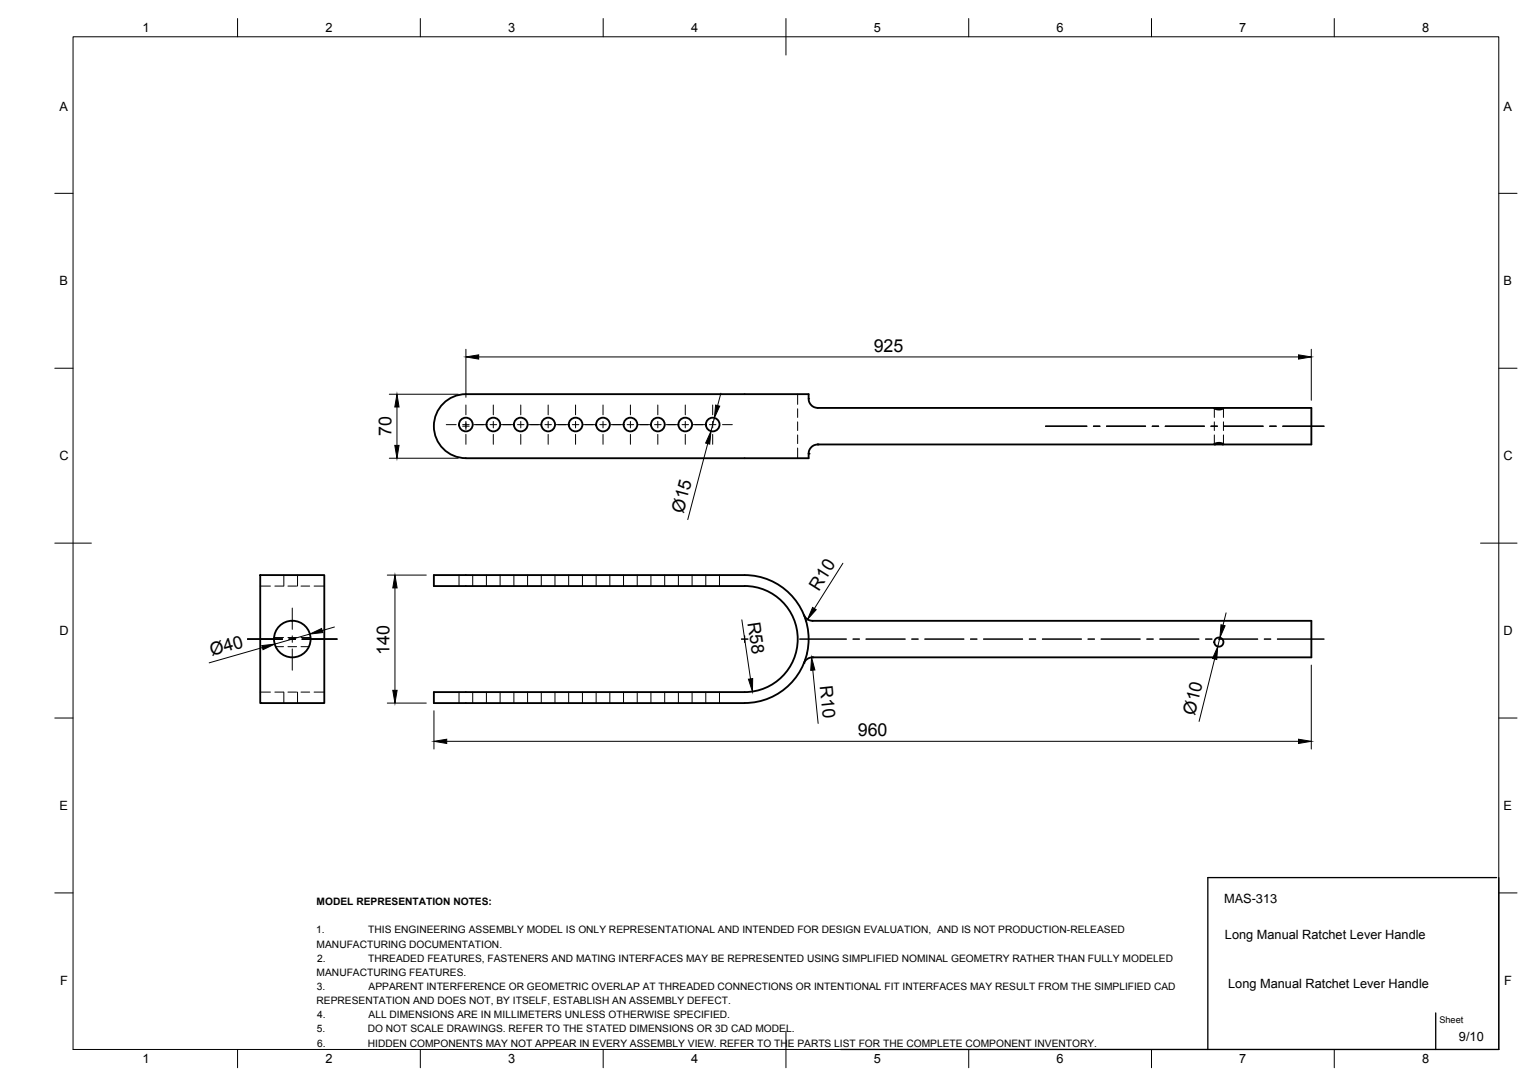
ISO-10303-21;
HEADER;
FILE_DESCRIPTION (('STEP AP214'),
    '1' );
FILE_NAME ('Long Manual Ratchet Lever Handle.step',
    '2026-10-06T09:36:00',
    ( '' ),
    ( '' ),
    'SwSTEP 2.0',
    'SolidWorks 2025',
    '' );
FILE_SCHEMA (( 'AUTOMOTIVE_DESIGN' ));
ENDSEC;

DATA;
#3=LINE ( 'NONE', #10333, #7200 ) ;
#5=EDGE_LOOP ( 'NONE', ( #11080, #1788 ) ) ;
#6=CARTESIAN_POINT ( 'NONE',  ( -384.9774416452893888, 80.69083648313058177, -144.6406486762352870 ) ) ;
#8=CARTESIAN_POINT ( 'NONE',  ( -374.9348459032029837, 78.20628728207141478, -105.0188168623670322 ) ) ;
#9=CARTESIAN_POINT ( 'NONE',  ( -305.0000000000000568, 81.99999999999995737, -89.68077099980384048 ) ) ;
#12=DIRECTION ( 'NONE',  ( -8.163404592832030268E-17, 1.000000000000000000, -0.000000000000000000 ) ) ;
#21=CARTESIAN_POINT ( 'NONE',  ( -824.1603064692799308, 83.67418067986842800, -144.6105757924095485 ) ) ;
#22=ADVANCED_FACE ( 'NONE', ( #9876 ), #2276, .F. ) ;
#24=CARTESIAN_POINT ( 'NONE',  ( -374.1619648394964770, 92.84764663444484256, -97.33358173750130504 ) ) ;
#35=CARTESIAN_POINT ( 'NONE',  ( -374.8624431792070482, 77.47276654782569949, -154.2594059479313842 ) ) ;
#36=CARTESIAN_POINT ( 'NONE',  ( -372.1683858186218004, 101.7385701426550071, -104.8071179324957569 ) ) ;
#42=LINE ( 'NONE', #11363, #8844 ) ;
#43=AXIS2_PLACEMENT_3D ( 'NONE', #1624, #5382, #1881 ) ;
#51=CARTESIAN_POINT ( 'NONE',  ( -379.1625717519825685, 101.9990905548760622, -123.9924296326342414 ) ) ;
#53=DIRECTION ( 'NONE',  ( -8.163404592832030268E-17, 1.000000000000000000, -0.000000000000000000 ) ) ;
#57=CARTESIAN_POINT ( 'NONE',  ( -370.6528479074003144, 106.2912024161782654, -136.2244394883228154 ) ) ;
#65=CARTESIAN_POINT ( 'NONE',  ( -365.0000000000000568, 81.99999999999997158, -124.6807709998038405 ) ) ;
#66=CARTESIAN_POINT ( 'NONE',  ( -119.9999999999999858, 12.00000000000001421, -126.4213562373086575 ) ) ;
#70=CARTESIAN_POINT ( 'NONE',  ( -384.9468357058332799, 80.02786880483864707, -144.5860799529720566 ) ) ;
#72=CARTESIAN_POINT ( 'NONE',  ( -374.8121035591796044, 76.80383275076532357, -95.25780428797004618 ) ) ;
#80=CARTESIAN_POINT ( 'NONE',  ( -97.49999999999998579, 24.00000000000001421, -126.4213562373088564 ) ) ;
#84=CARTESIAN_POINT ( 'NONE',  ( -384.0214413967224800, 73.66668219692796526, -106.4901515991773522 ) ) ;
#86=EDGE_CURVE ( 'NONE', #586, #9244, #5121, .T. ) ;
#90=VERTEX_POINT ( 'NONE', #4259 ) ;
#92=LINE ( 'NONE', #10358, #965 ) ;
#102=CARTESIAN_POINT ( 'NONE',  ( -383.2436296729866285, 93.11778785828077787, -108.0524282450768681 ) ) ;
#105=EDGE_CURVE ( 'NONE', #546, #9394, #11040, .T. ) ;
#111=DIRECTION ( 'NONE',  ( -8.163404592832030268E-17, 1.000000000000000000, -0.000000000000000000 ) ) ;
#120=EDGE_CURVE ( 'NONE', #2594, #3971, #5709, .T. ) ;
#121=EDGE_CURVE ( 'NONE', #609, #1988, #8932, .T. ) ;
#124=ORIENTED_EDGE ( 'NONE', *, *, #7991, .T. ) ;
#128=FACE_BOUND ( 'NONE', #2869, .T. ) ;
#130=CARTESIAN_POINT ( 'NONE',  ( -383.8870708247850985, 73.11411249519194655, -142.6104777306848916 ) ) ;
#132=CARTESIAN_POINT ( 'NONE',  ( -384.9021618238296583, 79.34260306531722051, -104.8553288783483453 ) ) ;
#141=CARTESIAN_POINT ( 'NONE',  ( -385.0078061158059768, 82.93686821115872476, -104.6668923901645769 ) ) ;
#143=EDGE_LOOP ( 'NONE', ( #3113, #5997, #4149, #12106, #10278, #5170, #6052 ) ) ;
#145=ORIENTED_EDGE ( 'NONE', *, *, #5842, .F. ) ;
#149=FACE_OUTER_BOUND ( 'NONE', #6887, .T. ) ;
#150=CIRCLE ( 'NONE', #8476, 7.500000000000007105 ) ;
#152=ORIENTED_EDGE ( 'NONE', *, *, #2859, .F. ) ;
#153=CARTESIAN_POINT ( 'NONE',  ( -374.9443013845391874, 79.15238586648754904, -154.5107090977903113 ) ) ;
#161=EDGE_CURVE ( 'NONE', #6627, #7697, #6700, .T. ) ;
#164=CARTESIAN_POINT ( 'NONE',  ( -150.0000000000000000, -9.213203435596451385, -126.4213562373084301 ) ) ;
#165=EDGE_CURVE ( 'NONE', #7498, #4712, #7501, .T. ) ;
#170=CARTESIAN_POINT ( 'NONE',  ( -371.2169330467067994, 104.7056300760318379, -109.5948443055706036 ) ) ;
#172=CARTESIAN_POINT ( 'NONE',  ( 1.414009460465297036E-14, -9.213203435596451385, -126.4213562373094959 ) ) ;
#174=CARTESIAN_POINT ( 'NONE',  ( -240.0000000000000000, 151.9999999999999716, -126.4213562373078190 ) ) ;
#179=ORIENTED_EDGE ( 'NONE', *, *, #161, .T. ) ;
#180=CYLINDRICAL_SURFACE ( 'NONE', #1475, 20.00000000000004619 ) ;
#181=CARTESIAN_POINT ( 'NONE',  ( -380.7070114274824846, 99.23877955377430737, -134.8374997946181111 ) ) ;
#183=EDGE_LOOP ( 'NONE', ( #1625, #2228, #7810, #4343, #5772, #11900, #7059 ) ) ;
#185=CARTESIAN_POINT ( 'NONE',  ( -384.7087986609971608, 86.59177257609081835, -144.1578396759514646 ) ) ;
#187=CARTESIAN_POINT ( 'NONE',  ( -382.1259332444888628, 67.82440028630135487, -110.5571689112878033 ) ) ;
#192=VERTEX_POINT ( 'NONE', #5981 ) ;
#200=CARTESIAN_POINT ( 'NONE',  ( -384.9575332945760806, 80.23676698716798228, -104.7563694268733059 ) ) ;
#204=CARTESIAN_POINT ( 'NONE',  ( -305.0000000000000568, 11.99999999999998224, -89.68077099980384048 ) ) ;
#210=DIRECTION ( 'NONE',  ( 3.061276722312011504E-17, -1.000000000000000000, 0.000000000000000000 ) ) ;
#211=CARTESIAN_POINT ( 'NONE',  ( -240.0000000000000000, 24.00000000000000711, -126.4213562373078190 ) ) ;
#218=EDGE_LOOP ( 'NONE', ( #11467, #11457 ) ) ;
#223=CIRCLE ( 'NONE', #7140, 7.500000000000007105 ) ;
#227=CARTESIAN_POINT ( 'NONE',  ( -820.5194676126008062, 82.43685310047841597, -104.6842045117117266 ) ) ;
#232=FACE_BOUND ( 'NONE', #2861, .T. ) ;
#233=VERTEX_POINT ( 'NONE', #6533 ) ;
#243=CARTESIAN_POINT ( 'NONE',  ( -383.7609474437092558, 91.40550212013970111, -142.3698073093449636 ) ) ;
#247=CARTESIAN_POINT ( 'NONE',  ( -384.0991065115986771, 74.01283611578425337, -143.0196247845297819 ) ) ;
#250=EDGE_LOOP ( 'NONE', ( #6658, #11800 ) ) ;
#263=ORIENTED_EDGE ( 'NONE', *, *, #5400, .T. ) ;
#270=ADVANCED_FACE ( 'NONE', ( #2701 ), #10246, .F. ) ;
#273=DIRECTION ( 'NONE',  ( -0.000000000000000000, -0.000000000000000000, -1.000000000000000000 ) ) ;
#283=EDGE_LOOP ( 'NONE', ( #6385, #2027 ) ) ;
#286=( BOUNDED_SURFACE ( )  B_SPLINE_SURFACE ( 3, 2, ( 
 ( #5085, #8801, #7187 ),
 ( #2485, #10957, #1263 ),
 ( #8857, #5024, #11650 ),
 ( #3170, #3727, #4408 ),
 ( #11016, #2547, #5517 ),
 ( #8178, #6322, #5324 ),
 ( #7317, #11945, #8318 ),
 ( #10089, #8249, #6509 ),
 ( #10030, #9093, #12007 ),
 ( #1688, #3526, #11218 ),
 ( #7251, #4472, #11082 ),
 ( #5581, #9355, #1623 ),
 ( #9160, #4606, #10151 ),
 ( #5381, #7377, #6262 ),
 ( #2741, #696, #632 ),
 ( #2607, #12145, #10219 ),
 ( #3462, #6382, #1561 ),
 ( #4667, #11150, #5445 ),
 ( #8445, #833, #9293 ),
 ( #9226, #767, #1818 ),
 ( #10279, #4542, #12077 ),
 ( #3587, #2673, #8382 ),
 ( #6448, #1756, #3659 ),
 ( #12203, #7433, #7499 ),
 ( #11272, #899, #10395 ),
 ( #1013, #1880, #10338 ),
 ( #9532, #6744, #8677 ),
 ( #2057, #5700, #5878 ),
 ( #7805, #8611, #130 ),
 ( #6810, #3848, #247 ),
 ( #5644, #3967, #9417 ),
 ( #1077, #4724, #2801 ),
 ( #8500, #5755, #10464 ),
 ( #4780, #6573, #7557 ),
 ( #9594, #5816, #8551 ),
 ( #2982, #6688, #4890 ),
 ( #953, #2119, #70 ),
 ( #1999, #7621, #6 ),
 ( #8730, #4035, #11511 ),
 ( #3782, #3908, #1938 ),
 ( #4834, #1139, #9657 ),
 ( #11329, #7682, #11389 ),
 ( #2928, #10521, #2870 ),
 ( #6630, #11451, #1198 ),
 ( #7737, #9474, #185 ),
 ( #10581, #3039, #4953 ),
 ( #11376, #2915, #12133 ),
 ( #2729, #1924, #3713 ),
 ( #5746, #7490, #5685 ),
 ( #6437, #6677, #10272 ),
 ( #11264, #5568, #10208 ),
 ( #9521, #1746, #2791 ),
 ( #8368, #11315, #11205 ),
 ( #3646, #5508, #1066 ),
 ( #9283, #5631, #1805 ),
 ( #6561, #1501, #821 ),
 ( #6498, #10325, #12064 ),
 ( #4766, #9405, #2854 ),
 ( #7611, #4713, #3773 ),
 ( #6620, #999, #8541 ),
 ( #57, #3836, #398 ),
 ( #9872, #8599, #11437 ) ),
 .UNSPECIFIED., .F., .F., .F. ) 
 B_SPLINE_SURFACE_WITH_KNOTS ( ( 4, 2, 2, 2, 2, 2, 2, 2, 2, 2, 2, 2, 2, 2, 2, 2, 2, 2, 2, 2, 2, 2, 2, 2, 2, 2, 2, 2, 2, 2, 4 ),
 ( 3, 3 ),
 ( 0.09449389133479987879, 0.1003997595432298551, 0.1063056277516598314, 0.1092585618558748195, 0.1107350289079823136, 0.1122114959600898076, 0.1181173641685197701, 0.1195938312206272502, 0.1210702982727347443, 0.1240232323769497325, 0.1269761664811647206, 0.1284526335332722147, 0.1299291005853797087, 0.1358349687938096850, 0.1387879028980246732, 0.1402643699501321672, 0.1417408370022396613, 0.1476467052106696376, 0.1491231722627771317, 0.1505996393148846257, 0.1535525734190996139, 0.1565055075233146020, 0.1594584416275295902, 0.1653643098359595387, 0.1683172439401744991, 0.1697937109922819932, 0.1712701780443894872, 0.1771760462528194635, 0.1801289803570344517, 0.1830819144612494398, 0.1889877826696794161 ),
 ( 0.000000000000000000, 1.000000000000000000 ),
 .UNSPECIFIED. ) 
 GEOMETRIC_REPRESENTATION_ITEM ( )  RATIONAL_B_SPLINE_SURFACE ( (
 ( 1.000000000000000000, 0.8172789612915526414, 1.000000000000000000),
 ( 1.000000000000000000, 0.8218272198189814359, 1.000000000000000000),
 ( 1.000000000000000000, 0.8252177520338900285, 1.000000000000000000),
 ( 1.000000000000000000, 0.8291640623197805704, 1.000000000000000000),
 ( 1.000000000000000000, 0.8296443862460527452, 1.000000000000000000),
 ( 1.000000000000000000, 0.8281763619574273871, 1.000000000000000000),
 ( 1.000000000000000000, 0.8273214979613470188, 1.000000000000000000),
 ( 1.000000000000000000, 0.8254906886306150327, 1.000000000000000000),
 ( 1.000000000000000000, 0.8247876722294519292, 1.000000000000000000),
 ( 1.000000000000000000, 0.8232192861295574149, 1.000000000000000000),
 ( 1.000000000000000000, 0.8223523569020266821, 1.000000000000000000),
 ( 1.000000000000000000, 0.8176244427683647675, 1.000000000000000000),
 ( 1.000000000000000000, 0.8125861978211987857, 1.000000000000000000),
 ( 1.000000000000000000, 0.8050068216217169947, 1.000000000000000000),
 ( 1.000000000000000000, 0.8034229420457332793, 1.000000000000000000),
 ( 1.000000000000000000, 0.8001526181735703069, 1.000000000000000000),
 ( 1.000000000000000000, 0.7984703186739749992, 1.000000000000000000),
 ( 1.000000000000000000, 0.7932997541396797914, 1.000000000000000000),
 ( 1.000000000000000000, 0.7896878191176920359, 1.000000000000000000),
 ( 1.000000000000000000, 0.7822263873999749650, 1.000000000000000000),
 ( 1.000000000000000000, 0.7783766572002538409, 1.000000000000000000),
 ( 1.000000000000000000, 0.7724948447777896243, 1.000000000000000000),
 ( 1.000000000000000000, 0.7705164146871855690, 1.000000000000000000),
 ( 1.000000000000000000, 0.7665366243600161278, 1.000000000000000000),
 ( 1.000000000000000000, 0.7645334732995007210, 1.000000000000000000),
 ( 1.000000000000000000, 0.7545994289160806723, 1.000000000000000000),
 ( 1.000000000000000000, 0.7468282588146691880, 1.000000000000000000),
 ( 1.000000000000000000, 0.7361158826353683127, 1.000000000000000000),
 ( 1.000000000000000000, 0.7327031703348744207, 1.000000000000000000),
 ( 1.000000000000000000, 0.7279177720675241714, 1.000000000000000000),
 ( 1.000000000000000000, 0.7263769756471946115, 1.000000000000000000),
 ( 1.000000000000000000, 0.7234575735669767083, 1.000000000000000000),
 ( 1.000000000000000000, 0.7220742453523991689, 1.000000000000000000),
 ( 1.000000000000000000, 0.7155655556167423992, 1.000000000000000000),
 ( 1.000000000000000000, 0.7116656400988581321, 1.000000000000000000),
 ( 1.000000000000000000, 0.7088249914908492100, 1.000000000000000000),
 ( 1.000000000000000000, 0.7083584775623817942, 1.000000000000000000),
 ( 1.000000000000000000, 0.7076383381209198076, 1.000000000000000000),
 ( 1.000000000000000000, 0.7073855737940044630, 1.000000000000000000),
 ( 1.000000000000000000, 0.7069609716970313151, 1.000000000000000000),
 ( 1.000000000000000000, 0.7071175024107954066, 1.000000000000000000),
 ( 1.000000000000000000, 0.7082797836801750790, 1.000000000000000000),
 ( 1.000000000000000000, 0.7092855318707916856, 1.000000000000000000),
 ( 1.000000000000000000, 0.7121081611133525113, 1.000000000000000000),
 ( 1.000000000000000000, 0.7139297788701386427, 1.000000000000000000),
 ( 1.000000000000000000, 0.7205123102341589592, 1.000000000000000000),
 ( 1.000000000000000000, 0.7262634879477153360, 1.000000000000000000),
 ( 1.000000000000000000, 0.7362377633225355433, 1.000000000000000000),
 ( 1.000000000000000000, 0.7397880641819555292, 1.000000000000000000),
 ( 1.000000000000000000, 0.7453704836958430224, 1.000000000000000000),
 ( 1.000000000000000000, 0.7472719429557758142, 1.000000000000000000),
 ( 1.000000000000000000, 0.7511059034608574825, 1.000000000000000000),
 ( 1.000000000000000000, 0.7530430930858292848, 1.000000000000000000),
 ( 1.000000000000000000, 0.7627925276597339321, 1.000000000000000000),
 ( 1.000000000000000000, 0.7707906794718482058, 1.000000000000000000),
 ( 1.000000000000000000, 0.7824407450661361452, 1.000000000000000000),
 ( 1.000000000000000000, 0.7862798113962640167, 1.000000000000000000),
 ( 1.000000000000000000, 0.7935920352645898790, 1.000000000000000000),
 ( 1.000000000000000000, 0.7970830763616314485, 1.000000000000000000),
 ( 1.000000000000000000, 0.8069453338637414541, 1.000000000000000000),
 ( 1.000000000000000000, 0.8127078027066928501, 1.000000000000000000),
 ( 1.000000000000000000, 0.8173438319342977154, 1.000000000000000000) ) ) 
 REPRESENTATION_ITEM ( '' )  SURFACE ( )  );
#288=AXIS2_PLACEMENT_3D ( 'NONE', #7289, #5491, #4381 ) ;
#290=CARTESIAN_POINT ( 'NONE',  ( -821.1548363108382773, 74.44610204637874062, -143.1996371447159788 ) ) ;
#294=CARTESIAN_POINT ( 'NONE',  ( -372.7969387542311210, 100.6399613739977497, -117.3710749709770198 ) ) ;
#297=FACE_BOUND ( 'NONE', #8922, .T. ) ;
#301=CARTESIAN_POINT ( 'NONE',  ( 7.500000000000022204, -9.213203435596451385, -126.4213562373094959 ) ) ;
#304=ORIENTED_EDGE ( 'NONE', *, *, #9166, .F. ) ;
#308=FACE_BOUND ( 'NONE', #6793, .T. ) ;
#311=DIRECTION ( 'NONE',  ( -1.000000000000000000, 0.000000000000000000, 0.000000000000000000 ) ) ;
#314=AXIS2_PLACEMENT_3D ( 'NONE', #7746, #6638, #6880 ) ;
#316=EDGE_LOOP ( 'NONE', ( #9146, #634 ) ) ;
#322=ORIENTED_EDGE ( 'NONE', *, *, #4849, .T. ) ;
#323=CYLINDRICAL_SURFACE ( 'NONE', #3336, 7.500000000000007105 ) ;
#324=CARTESIAN_POINT ( 'NONE',  ( -380.4203626278499542, 64.21146706504150359, -115.5204214313296376 ) ) ;
#330=DIRECTION ( 'NONE',  ( -1.000000000000000000, 0.000000000000000000, 0.000000000000000000 ) ) ;
#334=CIRCLE ( 'NONE', #5074, 57.99999999999999289 ) ;
#339=LINE ( 'NONE', #9047, #1075 ) ;
#342=EDGE_CURVE ( 'NONE', #12110, #8166, #11773, .T. ) ;
#351=AXIS2_PLACEMENT_3D ( 'NONE', #10311, #1910, #9449 ) ;
#352=DIRECTION ( 'NONE',  ( 0.000000000000000000, 0.000000000000000000, 1.000000000000000000 ) ) ;
#357=CIRCLE ( 'NONE', #7273, 7.499999999999992895 ) ;
#359=FACE_OUTER_BOUND ( 'NONE', #1203, .T. ) ;
#363=CARTESIAN_POINT ( 'NONE',  ( -375.0000000000000000, 81.99999999999995737, -89.68077099980384048 ) ) ;
#364=CARTESIAN_POINT ( 'NONE',  ( -374.9435208796285224, 79.09557628031252818, -94.85325544560421918 ) ) ;
#369=CARTESIAN_POINT ( 'NONE',  ( -90.00000000000000000, 152.0000000000000000, -126.4213562373088564 ) ) ;
#370=FACE_BOUND ( 'NONE', #3925, .T. ) ;
#373=CARTESIAN_POINT ( 'NONE',  ( -22.49999999999997868, -9.213203435596451385, -126.4213562373092685 ) ) ;
#379=ORIENTED_EDGE ( 'NONE', *, *, #11461, .F. ) ;
#380=ORIENTED_EDGE ( 'NONE', *, *, #161, .F. ) ;
#391=EDGE_CURVE ( 'NONE', #7319, #11283, #7095, .T. ) ;
#396=ORIENTED_EDGE ( 'NONE', *, *, #11359, .T. ) ;
#398=CARTESIAN_POINT ( 'NONE',  ( -380.0318359341034693, 100.5075656702939142, -132.3766003259852084 ) ) ;
#400=CYLINDRICAL_SURFACE ( 'NONE', #7484, 7.500000000000007105 ) ;
#401=EDGE_CURVE ( 'NONE', #10520, #8134, #578, .T. ) ;
#402=CARTESIAN_POINT ( 'NONE',  ( -180.0000000000000000, 12.00000000000001421, -126.4213562373082453 ) ) ;
#414=EDGE_CURVE ( 'NONE', #957, #11231, #4747, .T. ) ;
#419=CARTESIAN_POINT ( 'NONE',  ( -373.3204616456844747, 97.25197993938448349, -149.1095482086399784 ) ) ;
#442=CARTESIAN_POINT ( 'NONE',  ( -90.00000000000000000, 139.9999999999999716, -126.4213562373088564 ) ) ;
#448=DIRECTION ( 'NONE',  ( -1.000000000000000000, 0.000000000000000000, 0.000000000000000000 ) ) ;
#449=AXIS2_PLACEMENT_3D ( 'NONE', #6036, #2435, #448 ) ;
#451=CIRCLE ( 'NONE', #3416, 7.500000000000007105 ) ;
#466=CARTESIAN_POINT ( 'NONE',  ( -824.1545993022709808, 83.67440335600066703, -104.7509849144497736 ) ) ;
#469=LINE ( 'NONE', #4263, #6510 ) ;
#475=VECTOR ( 'NONE', #10063, 1000.000000000000000 ) ;
#478=ADVANCED_FACE ( 'NONE', ( #7705, #4803, #8575, #5910, #10363, #9558, #10543, #5725, #8699, #6657, #2827 ), #11414, .F. ) ;
#479=DIRECTION ( 'NONE',  ( 1.000000000000000000, 1.486905836551548832E-16, -0.000000000000000000 ) ) ;
#483=CIRCLE ( 'NONE', #3067, 7.500000000000007105 ) ;
#488=CARTESIAN_POINT ( 'NONE',  ( -374.5655304648819879, 89.79463081985890938, -153.3305951811361751 ) ) ;
#495=VERTEX_POINT ( 'NONE', #7765 ) ;
#496=EDGE_CURVE ( 'NONE', #546, #9681, #11781, .T. ) ;
#501=CARTESIAN_POINT ( 'NONE',  ( -379.1619848709567577, 102.0000000000000284, -123.4679443962072725 ) ) ;
#503=AXIS2_PLACEMENT_3D ( 'NONE', #6514, #3590, #1821 ) ;
#514=CARTESIAN_POINT ( 'NONE',  ( -374.8923245633905026, 85.92087493068839876, -95.01038614168759011 ) ) ;
#516=DIRECTION ( 'NONE',  ( 1.000000000000000000, 0.000000000000000000, 0.000000000000000000 ) ) ;
#517=CARTESIAN_POINT ( 'NONE',  ( -374.9998907128388623, 83.71581840400844499, -94.68015511488202662 ) ) ;
#518=ORIENTED_EDGE ( 'NONE', *, *, #8104, .T. ) ;
#521=ORIENTED_EDGE ( 'NONE', *, *, #11514, .T. ) ;
#528=DIRECTION ( 'NONE',  ( -8.163404592832031500E-17, 1.000000000000000000, 0.000000000000000000 ) ) ;
#529=CARTESIAN_POINT ( 'NONE',  ( -119.9999999999999858, 24.00000000000001421, -126.4213562373086575 ) ) ;
#531=CARTESIAN_POINT ( 'NONE',  ( -819.1462522098552199, 76.91297450996658824, -144.0236343770278609 ) ) ;
#536=ORIENTED_EDGE ( 'NONE', *, *, #1166, .F. ) ;
#537=FACE_OUTER_BOUND ( 'NONE', #8170, .T. ) ;
#542=EDGE_CURVE ( 'NONE', #9452, #8983, #6330, .T. ) ;
#546=VERTEX_POINT ( 'NONE', #9798 ) ;
#551=CARTESIAN_POINT ( 'NONE',  ( -370.0721644750066730, 107.8006199747635492, -130.5475387910841221 ) ) ;
#553=ADVANCED_FACE ( 'NONE', ( #5206 ), #2432, .T. ) ;
#555=DIRECTION ( 'NONE',  ( -8.163404592832030268E-17, 1.000000000000000000, -0.000000000000000000 ) ) ;
#563=ORIENTED_EDGE ( 'NONE', *, *, #496, .T. ) ;
#568=AXIS2_PLACEMENT_3D ( 'NONE', #5738, #2909, #4137 ) ;
#578=CIRCLE ( 'NONE', #1190, 7.500000000000007105 ) ;
#582=DIRECTION ( 'NONE',  ( 1.776356839400250465E-15, 0.000000000000000000, 1.000000000000000000 ) ) ;
#586=VERTEX_POINT ( 'NONE', #7135 ) ;
#589=DIRECTION ( 'NONE',  ( 1.000000000000000000, 2.040851148208007875E-17, 0.000000000000000000 ) ) ;
#590=CARTESIAN_POINT ( 'NONE',  ( -89.99999999999998579, -9.213203435596451385, -126.4213562373088564 ) ) ;
#591=ORIENTED_EDGE ( 'NONE', *, *, #3649, .T. ) ;
#597=CARTESIAN_POINT ( 'NONE',  ( -828.7636281597782499, 77.85463023298294161, -144.2471423470011018 ) ) ;
#606=FACE_OUTER_BOUND ( 'NONE', #11571, .T. ) ;
#609=VERTEX_POINT ( 'NONE', #9044 ) ;
#619=ORIENTED_EDGE ( 'NONE', *, *, #2215, .T. ) ;
#620=DIRECTION ( 'NONE',  ( -8.163404592832030268E-17, 1.000000000000000000, -0.000000000000000000 ) ) ;
#629=AXIS2_PLACEMENT_3D ( 'NONE', #5807, #4770, #10387 ) ;
#632=CARTESIAN_POINT ( 'NONE',  ( -380.5094386830780877, 64.38196187857104746, -134.1524419411843212 ) ) ;
#633=CARTESIAN_POINT ( 'NONE',  ( -29.99999999999998579, -9.213203435596451385, -126.4213562373092685 ) ) ;
#634=ORIENTED_EDGE ( 'NONE', *, *, #105, .F. ) ;
#637=EDGE_LOOP ( 'NONE', ( #8862, #9287, #8745, #1050 ) ) ;
#642=DIRECTION ( 'NONE',  ( 1.000000000000000000, 0.000000000000000000, 0.000000000000000000 ) ) ;
#648=CARTESIAN_POINT ( 'NONE',  ( -379.7887390581964837, 110.4014878146373633, -134.3428354745942102 ) ) ;
#652=CARTESIAN_POINT ( 'NONE',  ( -59.99999999999998579, -9.213203435596451385, -126.4213562373090696 ) ) ;
#654=EDGE_CURVE ( 'NONE', #2078, #6153, #6149, .T. ) ;
#658=CARTESIAN_POINT ( 'NONE',  ( -828.3259789886573117, 76.46577308275197993, -105.4592182070448416 ) ) ;
#666=EDGE_LOOP ( 'NONE', ( #1393, #6344, #2255, #9869 ) ) ;
#696=CARTESIAN_POINT ( 'NONE',  ( -373.1983853544816725, 64.95592079649878769, -135.2209821354010728 ) ) ;
#697=CYLINDRICAL_SURFACE ( 'NONE', #6175, 7.499999999999992895 ) ;
#698=EDGE_LOOP ( 'NONE', ( #3165, #3081, #2133, #7527, #1551 ) ) ;
#700=AXIS2_PLACEMENT_3D ( 'NONE', #10293, #12095, #7515 ) ;
#708=EDGE_CURVE ( 'NONE', #4719, #2602, #5527, .T. ) ;
#719=CARTESIAN_POINT ( 'NONE',  ( -30.00000000000000000, 139.9999999999999716, -126.4213562373092685 ) ) ;
#726=CARTESIAN_POINT ( 'NONE',  ( -369.8747838094790268, 55.70677269066278825, -126.1647431307883522 ) ) ;
#728=DIRECTION ( 'NONE',  ( 1.000000000000000000, 0.000000000000000000, 0.000000000000000000 ) ) ;
#735=DIRECTION ( 'NONE',  ( 0.000000000000000000, 1.000000000000000000, -0.000000000000000000 ) ) ;
#741=DIRECTION ( 'NONE',  ( 1.000000000000000000, 1.486905836551548832E-16, -0.000000000000000000 ) ) ;
#758=ORIENTED_EDGE ( 'NONE', *, *, #1083, .F. ) ;
#767=CARTESIAN_POINT ( 'NONE',  ( -373.7506463163484796, 67.50546400631965582, -138.5607443211070802 ) ) ;
#774=DIRECTION ( 'NONE',  ( 3.061276722312011504E-17, -1.000000000000000000, 0.000000000000000000 ) ) ;
#784=CARTESIAN_POINT ( 'NONE',  ( -369.8980370199456047, 108.2344238686749520, -123.1401886717858787 ) ) ;
#785=ORIENTED_EDGE ( 'NONE', *, *, #9267, .F. ) ;
#787=VECTOR ( 'NONE', #1857, 1000.000000000000000 ) ;
#794=CARTESIAN_POINT ( 'NONE',  ( -820.7525053003647599, 74.71879621637245350, -106.0522004026985456 ) ) ;
#801=CARTESIAN_POINT ( 'NONE',  ( -374.4786324000669424, 91.82513850978268977, -107.1885437437087063 ) ) ;
#805=DIRECTION ( 'NONE',  ( -1.000000000000000000, 0.000000000000000000, 0.000000000000000000 ) ) ;
#817=CARTESIAN_POINT ( 'NONE',  ( -82.49999999999997158, -9.213203435596451385, -126.4213562373088564 ) ) ;
#818=VERTEX_POINT ( 'NONE', #8260 ) ;
#820=LINE ( 'NONE', #1865, #6878 ) ;
#821=CARTESIAN_POINT ( 'NONE',  ( -381.5603242327452449, 97.47709203580956228, -137.3647392459991750 ) ) ;
#824=EDGE_CURVE ( 'NONE', #11283, #7319, #1411, .T. ) ;
#828=AXIS2_PLACEMENT_3D ( 'NONE', #6958, #5155, #8814 ) ;
#833=CARTESIAN_POINT ( 'NONE',  ( -373.5661612086483387, 66.59315941246912018, -137.5313104353387530 ) ) ;
#836=DIRECTION ( 'NONE',  ( -1.000000000000000000, 0.000000000000000000, 0.000000000000000000 ) ) ;
#845=DIRECTION ( 'NONE',  ( 2.040851148208007875E-17, -1.000000000000000000, -0.000000000000000000 ) ) ;
#846=VECTOR ( 'NONE', #8160, 1000.000000000000000 ) ;
#847=CIRCLE ( 'NONE', #2211, 7.500000000000007105 ) ;
#849=ORIENTED_EDGE ( 'NONE', *, *, #4932, .F. ) ;
#851=CARTESIAN_POINT ( 'NONE',  ( -370.4631672708575252, 106.7912974028927806, -114.8027370444668662 ) ) ;
#855=CARTESIAN_POINT ( 'NONE',  ( -187.5000000000000000, 24.00000000000001421, -126.4213562373082453 ) ) ;
#859=AXIS2_PLACEMENT_3D ( 'NONE', #211, #8634, #7891 ) ;
#860=EDGE_CURVE ( 'NONE', #3022, #6536, #1699, .T. ) ;
#861=CARTESIAN_POINT ( 'NONE',  ( -823.4970567115291260, 73.67398878492905112, -106.4962298347509631 ) ) ;
#863=CARTESIAN_POINT ( 'NONE',  ( -826.3639150177590409, 74.35254223074673519, -143.1619793993633323 ) ) ;
#864=VERTEX_POINT ( 'NONE', #11160 ) ;
#865=CARTESIAN_POINT ( 'NONE',  ( -372.8682051073146226, 64.83784294256510350, -147.4127590854037635 ) ) ;
#866=CARTESIAN_POINT ( 'NONE',  ( -384.1845455826150442, 89.69765040021600555, -106.1749927342177102 ) ) ;
#876=LINE ( 'NONE', #8424, #1553 ) ;
#878=CARTESIAN_POINT ( 'NONE',  ( -369.9630775916107268, 108.0732521340322876, -120.6787736983387163 ) ) ;
#899=CARTESIAN_POINT ( 'NONE',  ( -374.1450238171013893, 69.75518729278782359, -140.5780087988560183 ) ) ;
#903=EDGE_CURVE ( 'NONE', #7035, #9732, #8909, .T. ) ;
#905=AXIS2_PLACEMENT_3D ( 'NONE', #9527, #2866, #1994 ) ;
#917=CARTESIAN_POINT ( 'NONE',  ( -373.0711960171485657, 98.34294693636040563, -101.1726803376526505 ) ) ;
#921=DIRECTION ( 'NONE',  ( 0.000000000000000000, -0.9464175275073136717, 0.3229456047493806103 ) ) ;
#922=CARTESIAN_POINT ( 'NONE',  ( -828.8285638327206470, 78.34605190446892209, -105.0145692953448133 ) ) ;
#925=EDGE_LOOP ( 'NONE', ( #10478, #7807, #5815, #9444 ) ) ;
#932=AXIS2_PLACEMENT_3D ( 'NONE', #9914, #5152, #9977 ) ;
#945=VECTOR ( 'NONE', #10974, 1000.000000000000000 ) ;
#946=ORIENTED_EDGE ( 'NONE', *, *, #12081, .T. ) ;
#952=MECHANICAL_DESIGN_GEOMETRIC_PRESENTATION_REPRESENTATION('',(#1937),#2926);
#953=CARTESIAN_POINT ( 'NONE',  ( -374.9534812425817449, 79.41157780634799224, -154.5387344296071319 ) ) ;
#957=VERTEX_POINT ( 'NONE', #3052 ) ;
#958=CIRCLE ( 'NONE', #351, 7.500000000000007105 ) ;
#960=CARTESIAN_POINT ( 'NONE',  ( -97.49999999999998579, -9.213203435596451385, -126.4213562373088564 ) ) ;
#965=VECTOR ( 'NONE', #2823, 1000.000000000000000 ) ;
#966=VERTEX_POINT ( 'NONE', #80 ) ;
#970=CARTESIAN_POINT ( 'NONE',  ( -369.9251870295186677, 108.1672116062914029, -127.1279719650820255 ) ) ;
#973=DIRECTION ( 'NONE',  ( -8.163404592832030268E-17, 1.000000000000000000, -0.000000000000000000 ) ) ;
#976=AXIS2_PLACEMENT_3D ( 'NONE', #9716, #10818, #2236 ) ;
#979=CARTESIAN_POINT ( 'NONE',  ( -150.0000000000000000, -9.213203435596451385, -126.4213562373084301 ) ) ;
#981=CARTESIAN_POINT ( 'NONE',  ( -210.0000000000000000, -9.213203435596478030, -126.4213562373080180 ) ) ;
#996=DIRECTION ( 'NONE',  ( -8.163404592832030268E-17, 1.000000000000000000, -0.000000000000000000 ) ) ;
#999=CARTESIAN_POINT ( 'NONE',  ( -373.1039460868908009, 99.45530451436835051, -134.6103044504524462 ) ) ;
#1011=FACE_BOUND ( 'NONE', #10350, .T. ) ;
#1013=CARTESIAN_POINT ( 'NONE',  ( -373.1558531919824873, 65.98301015230569533, -148.5292176372442725 ) ) ;
#1014=EDGE_CURVE ( 'NONE', #11690, #11084, #1599, .T. ) ;
#1017=CYLINDRICAL_SURFACE ( 'NONE', #5268, 7.499999999999992895 ) ;
#1018=AXIS2_PLACEMENT_3D ( 'NONE', #7016, #1338, #5969 ) ;
#1022=CYLINDRICAL_SURFACE ( 'NONE', #4880, 7.500000000000007994 ) ;
#1027=ORIENTED_EDGE ( 'NONE', *, *, #3586, .T. ) ;
#1029=CARTESIAN_POINT ( 'NONE',  ( -826.3405481598703091, 83.00984762678743323, -144.6560901833811670 ) ) ;
#1032=CARTESIAN_POINT ( 'NONE',  ( -370.7906933011090587, 105.9194442196002797, -112.1115210325544211 ) ) ;
#1044=AXIS2_PLACEMENT_3D ( 'NONE', #7346, #6420, #10190 ) ;
#1046=DIRECTION ( 'NONE',  ( 0.000000000000000000, 1.000000000000000000, -0.000000000000000000 ) ) ;
#1047=CARTESIAN_POINT ( 'NONE',  ( -373.3860983059685168, 96.94888192596226872, -100.0157719451421201 ) ) ;
#1050=ORIENTED_EDGE ( 'NONE', *, *, #6377, .F. ) ;
#1058=LINE ( 'NONE', #8589, #4412 ) ;
#1061=CARTESIAN_POINT ( 'NONE',  ( -379.2435172475073841, 101.8653349591487398, -122.0127727988336233 ) ) ;
#1062=DIRECTION ( 'NONE',  ( -8.163404592832031500E-17, 1.000000000000000000, 0.000000000000000000 ) ) ;
#1063=CARTESIAN_POINT ( 'NONE',  ( -187.5000000000000000, -9.213203435596478030, -126.4213562373082453 ) ) ;
#1064=ORIENTED_EDGE ( 'NONE', *, *, #2859, .T. ) ;
#1066=CARTESIAN_POINT ( 'NONE',  ( -382.5082707561835491, 95.24935193720608595, -139.7187524817161659 ) ) ;
#1073=DIRECTION ( 'NONE',  ( 1.000000000000000000, 8.163404592832031500E-17, 0.000000000000000000 ) ) ;
#1075=VECTOR ( 'NONE', #9864, 1000.000000000000000 ) ;
#1077=CARTESIAN_POINT ( 'NONE',  ( -374.3833522074543794, 72.72018747391939542, -152.7479631189390830 ) ) ;
#1078=DIRECTION ( 'NONE',  ( -1.000000000000000000, 0.000000000000000000, 0.000000000000000000 ) ) ;
#1079=CARTESIAN_POINT ( 'NONE',  ( -372.7333679680364753, 64.32814225526269070, -102.4919576850857936 ) ) ;
#1080=LINE ( 'NONE', #3911, #7467 ) ;
#1083=EDGE_CURVE ( 'NONE', #6536, #957, #334, .T. ) ;
#1084=VECTOR ( 'NONE', #3811, 1000.000000000000000 ) ;
#1090=ORIENTED_EDGE ( 'NONE', *, *, #6921, .F. ) ;
#1099=CARTESIAN_POINT ( 'NONE',  ( -119.9999999999999858, 12.00000000000001421, -126.4213562373086575 ) ) ;
#1107=ADVANCED_FACE ( 'NONE', ( #5426, #10197 ), #7355, .T. ) ;
#1108=ORIENTED_EDGE ( 'NONE', *, *, #8570, .F. ) ;
#1120=CARTESIAN_POINT ( 'NONE',  ( -379.3756478403909682, 101.6476682939905629, -120.7185890014945784 ) ) ;
#1121=EDGE_CURVE ( 'NONE', #818, #12110, #7480, .T. ) ;
#1123=CARTESIAN_POINT ( 'NONE',  ( -60.00000000000000000, 152.0000000000000000, -126.4213562373090696 ) ) ;
#1124=ORIENTED_EDGE ( 'NONE', *, *, #4496, .F. ) ;
#1128=DIRECTION ( 'NONE',  ( 0.000000000000000000, 0.000000000000000000, 1.000000000000000000 ) ) ;
#1132=DIRECTION ( 'NONE',  ( -8.163404592832030268E-17, 1.000000000000000000, -0.000000000000000000 ) ) ;
#1136=DIRECTION ( 'NONE',  ( -1.000000000000000000, -2.040851148208007875E-17, 0.000000000000000000 ) ) ;
#1138=ORIENTED_EDGE ( 'NONE', *, *, #11671, .T. ) ;
#1139=CARTESIAN_POINT ( 'NONE',  ( -374.9999469826531140, 82.55142442433661643, -144.6804108797159643 ) ) ;
#1151=ORIENTED_EDGE ( 'NONE', *, *, #496, .F. ) ;
#1152=FACE_OUTER_BOUND ( 'NONE', #3781, .T. ) ;
#1157=EDGE_LOOP ( 'NONE', ( #5522, #946 ) ) ;
#1166=EDGE_CURVE ( 'NONE', #7292, #12134, #2810, .T. ) ;
#1170=ORIENTED_EDGE ( 'NONE', *, *, #4570, .T. ) ;
#1190=AXIS2_PLACEMENT_3D ( 'NONE', #8519, #10425, #3809 ) ;
#1192=VERTEX_POINT ( 'NONE', #5559 ) ;
#1193=CARTESIAN_POINT ( 'NONE',  ( -142.5000000000000000, 24.00000000000001421, -126.4213562373084301 ) ) ;
#1195=CARTESIAN_POINT ( 'NONE',  ( -382.8391312933034669, 94.32133009973502169, -140.4452862510830755 ) ) ;
#1198=CARTESIAN_POINT ( 'NONE',  ( -384.7868575475719695, 85.94460086465754500, -144.2989652200420494 ) ) ;
#1200=CARTESIAN_POINT ( 'NONE',  ( -374.6039973053199788, 73.23368555401432900, -106.6028248502465061 ) ) ;
#1203=EDGE_LOOP ( 'NONE', ( #10575, #3913, #8610, #5820 ) ) ;
#1204=ORIENTED_EDGE ( 'NONE', *, *, #8707, .F. ) ;
#1208=EDGE_LOOP ( 'NONE', ( #11716, #6844, #396, #5185 ) ) ;
#1209=CARTESIAN_POINT ( 'NONE',  ( -384.5582068021247437, 87.62753060213235301, -105.4794641167554232 ) ) ;
#1212=EDGE_LOOP ( 'NONE', ( #8401, #12199, #1064, #4026 ) ) ;
#1222=VECTOR ( 'NONE', #11804, 1000.000000000000000 ) ;
#1229=EDGE_CURVE ( 'NONE', #6950, #4621, #9334, .T. ) ;
#1233=VERTEX_POINT ( 'NONE', #1916 ) ;
#1235=CARTESIAN_POINT ( 'NONE',  ( -819.4838385048373084, 81.17047855582150362, -104.6961160549175531 ) ) ;
#1250=FACE_BOUND ( 'NONE', #218, .T. ) ;
#1252=FACE_OUTER_BOUND ( 'NONE', #4826, .T. ) ;
#1260=DIRECTION ( 'NONE',  ( -8.163404592832030268E-17, 1.000000000000000000, -0.000000000000000000 ) ) ;
#1263=CARTESIAN_POINT ( 'NONE',  ( -379.5535208569121437, 62.65259614875188987, -119.4499276052048771 ) ) ;
#1275=DIRECTION ( 'NONE',  ( -1.000000000000000000, 0.000000000000000000, 0.000000000000000000 ) ) ;
#1276=UNCERTAINTY_MEASURE_WITH_UNIT (LENGTH_MEASURE( 1.000000000000000082E-05 ), #10584, 'distance_accuracy_value', 'NONE');
#1277=ADVANCED_FACE ( 'NONE', ( #8533 ), #3766, .F. ) ;
#1279=DIRECTION ( 'NONE',  ( -1.000000000000000000, 0.000000000000000000, 0.000000000000000000 ) ) ;
#1294=CARTESIAN_POINT ( 'NONE',  ( -305.0000000000000568, 81.99999999999995737, -89.68077099980384048 ) ) ;
#1295=CARTESIAN_POINT ( 'NONE',  ( -67.50000000000000000, 139.9999999999999716, -126.4213562373090696 ) ) ;
#1298=DIRECTION ( 'NONE',  ( 1.000000000000000000, 0.000000000000000000, 0.000000000000000000 ) ) ;
#1302=DIRECTION ( 'NONE',  ( 1.000000000000000000, 0.000000000000000000, -0.000000000000000000 ) ) ;
#1309=EDGE_LOOP ( 'NONE', ( #11192, #9487, #5444, #2692 ) ) ;
#1313=DIRECTION ( 'NONE',  ( 2.040851148208007875E-17, -1.000000000000000000, -0.000000000000000000 ) ) ;
#1316=EDGE_CURVE ( 'NONE', #9732, #7035, #847, .T. ) ;
#1318=ORIENTED_EDGE ( 'NONE', *, *, #10928, .F. ) ;
#1324=CIRCLE ( 'NONE', #7436, 7.500000000000007105 ) ;
#1325=FACE_OUTER_BOUND ( 'NONE', #1959, .T. ) ;
#1327=ORIENTED_EDGE ( 'NONE', *, *, #2177, .F. ) ;
#1338=DIRECTION ( 'NONE',  ( -1.000000000000000000, -1.486905836551548832E-16, 0.000000000000000000 ) ) ;
#1344=EDGE_CURVE ( 'NONE', #233, #4125, #7080, .T. ) ;
#1352=CARTESIAN_POINT ( 'NONE',  ( -826.0484035456422589, 83.16661265238070655, -104.7144245788473000 ) ) ;
#1354=CARTESIAN_POINT ( 'NONE',  ( -373.2899463707186669, 98.65819193945954169, -113.5174344538613411 ) ) ;
#1356=VECTOR ( 'NONE', #973, 1000.000000000000000 ) ;
#1358=DIRECTION ( 'NONE',  ( -8.163404592832030268E-17, 1.000000000000000000, -0.000000000000000000 ) ) ;
#1362=CARTESIAN_POINT ( 'NONE',  ( -374.6494996980943597, 74.87479940665586753, -95.76181135420617352 ) ) ;
#1364=CIRCLE ( 'NONE', #11242, 7.500000000000020428 ) ;
#1366=CARTESIAN_POINT ( 'NONE',  ( -383.3184125885782692, 71.07417258413192940, -141.4727867585951344 ) ) ;
#1368=CARTESIAN_POINT ( 'NONE',  ( -217.5000000000000000, 24.00000000000000711, -126.4213562373080180 ) ) ;
#1371=CARTESIAN_POINT ( 'NONE',  ( -210.0000000000000000, -9.213203435596478030, -126.4213562373080180 ) ) ;
#1373=AXIS2_PLACEMENT_3D ( 'NONE', #6165, #1466, #352 ) ;
#1380=DIRECTION ( 'NONE',  ( -1.000000000000000000, 0.000000000000000000, 0.000000000000000000 ) ) ;
#1385=ORIENTED_EDGE ( 'NONE', *, *, #6553, .F. ) ;
#1393=ORIENTED_EDGE ( 'NONE', *, *, #4461, .F. ) ;
#1395=CARTESIAN_POINT ( 'NONE',  ( -370.4431240880616656, 57.15653990293294839, -114.9924028573224035 ) ) ;
#1407=EDGE_CURVE ( 'NONE', #11206, #8134, #1058, .T. ) ;
#1408=ADVANCED_FACE ( 'NONE', ( #7660 ), #11430, .F. ) ;
#1411=CIRCLE ( 'NONE', #8337, 7.500000000000007105 ) ;
#1418=EDGE_CURVE ( 'NONE', #8166, #12110, #10504, .T. ) ;
#1420=CARTESIAN_POINT ( 'NONE',  ( -202.4999999999999716, 151.9999999999999716, -126.4213562373080180 ) ) ;
#1421=CARTESIAN_POINT ( 'NONE',  ( -374.0142209343122772, 70.27728921848439825, -97.82681790556920021 ) ) ;
#1427=CARTESIAN_POINT ( 'NONE',  ( -379.7840584701665421, 63.05619850801249981, -131.1209148564447275 ) ) ;
#1432=VECTOR ( 'NONE', #8423, 1000.000000000000000 ) ;
#1435=AXIS2_PLACEMENT_3D ( 'NONE', #5645, #4409, #4607 ) ;
#1439=DIRECTION ( 'NONE',  ( -1.000000000000000000, 0.000000000000000000, 0.000000000000000000 ) ) ;
#1441=CARTESIAN_POINT ( 'NONE',  ( -67.49999999999998579, 12.00000000000001421, -126.4213562373090696 ) ) ;
#1442=CIRCLE ( 'NONE', #9353, 7.500000000000007105 ) ;
#1447=ORIENTED_EDGE ( 'NONE', *, *, #5229, .T. ) ;
#1449=CARTESIAN_POINT ( 'NONE',  ( -372.7937968025706255, 63.34872752675727270, -117.4098597798456041 ) ) ;
#1451=CARTESIAN_POINT ( 'NONE',  ( -270.0000000000000000, 151.9999999999999716, -126.4213562373076059 ) ) ;
#1461=VECTOR ( 'NONE', #6301, 1000.000000000000000 ) ;
#1464=AXIS2_PLACEMENT_3D ( 'NONE', #6953, #10721, #7642 ) ;
#1466=DIRECTION ( 'NONE',  ( 0.000000000000000000, 1.000000000000000000, -0.000000000000000000 ) ) ;
#1467=CARTESIAN_POINT ( 'NONE',  ( -305.0000000000000568, 151.9999999999999716, -159.6807709998038547 ) ) ;
#1475=AXIS2_PLACEMENT_3D ( 'NONE', #65, #3902, #8672 ) ;
#1478=DIRECTION ( 'NONE',  ( -8.163404592832030268E-17, 1.000000000000000000, -0.000000000000000000 ) ) ;
#1479=CARTESIAN_POINT ( 'NONE',  ( -373.6864081855313202, 68.44581660449321703, -98.94085437915049397 ) ) ;
#1489=CYLINDRICAL_SURFACE ( 'NONE', #11185, 7.500000000000007105 ) ;
#1491=CARTESIAN_POINT ( 'NONE',  ( 0.000000000000000000, 152.0000000000000000, -89.68077099980384048 ) ) ;
#1492=CYLINDRICAL_SURFACE ( 'NONE', #11425, 35.00000000000000000 ) ;
#1497=EDGE_LOOP ( 'NONE', ( #11987, #7229, #521, #8305 ) ) ;
#1501=CARTESIAN_POINT ( 'NONE',  ( -373.7456202422138176, 96.52126932011218230, -138.5319469839025714 ) ) ;
#1502=FACE_OUTER_BOUND ( 'NONE', #6460, .T. ) ;
#1511=ORIENTED_EDGE ( 'NONE', *, *, #12140, .F. ) ;
#1512=CARTESIAN_POINT ( 'NONE',  ( -150.0000000000000000, 24.00000000000001421, -126.4213562373084301 ) ) ;
#1519=CIRCLE ( 'NONE', #9424, 35.00000000000000000 ) ;
#1524=DIRECTION ( 'NONE',  ( -8.163404592832030268E-17, 1.000000000000000000, -0.000000000000000000 ) ) ;
#1526=CARTESIAN_POINT ( 'NONE',  ( -820.7495229154725394, 74.72132575352334527, -143.3103177350645296 ) ) ;
#1530=LINE ( 'NONE', #11678, #9648 ) ;
#1531=DIRECTION ( 'NONE',  ( -3.061276722312011504E-17, 1.000000000000000000, -0.000000000000000000 ) ) ;
#1532=ORIENTED_EDGE ( 'NONE', *, *, #10312, .T. ) ;
#1535=DIRECTION ( 'NONE',  ( -1.000000000000000000, 0.000000000000000000, 0.000000000000000000 ) ) ;
#1537=CARTESIAN_POINT ( 'NONE',  ( -370.5981920676458685, 57.56502298018414621, -113.6242979122189922 ) ) ;
#1547=CARTESIAN_POINT ( 'NONE',  ( -363.0000000000000568, 81.99999999999995737, -89.68077099980384048 ) ) ;
#1550=DIRECTION ( 'NONE',  ( -1.000000000000000000, 0.000000000000000000, 0.000000000000000000 ) ) ;
#1551=ORIENTED_EDGE ( 'NONE', *, *, #2991, .T. ) ;
#1553=VECTOR ( 'NONE', #3704, 1000.000000000000000 ) ;
#1560=EDGE_CURVE ( 'NONE', #9452, #495, #3946, .T. ) ;
#1561=CARTESIAN_POINT ( 'NONE',  ( -380.7611941007019141, 64.86892148911482536, -135.0070643092065836 ) ) ;
#1562=CARTESIAN_POINT ( 'NONE',  ( -381.5042408296175722, 97.59833250969687413, -112.1498553144568717 ) ) ;
#1565=DIRECTION ( 'NONE',  ( 0.000000000000000000, 0.000000000000000000, 1.000000000000000000 ) ) ;
#1568=CARTESIAN_POINT ( 'NONE',  ( -180.0000000000000000, -9.213203435596478030, -126.4213562373082453 ) ) ;
#1569=AXIS2_PLACEMENT_3D ( 'NONE', #11542, #273, #10607 ) ;
#1573=CARTESIAN_POINT ( 'NONE',  ( 7.500000000000020428, 12.00000000000001776, -126.4213562373094959 ) ) ;
#1575=CARTESIAN_POINT ( 'NONE',  ( -385.0247828397638159, 81.99275599918267687, -104.6365852498861102 ) ) ;
#1584=DIRECTION ( 'NONE',  ( -0.000000000000000000, -0.000000000000000000, 1.000000000000000000 ) ) ;
#1597=ORIENTED_EDGE ( 'NONE', *, *, #6226, .T. ) ;
#1599=LINE ( 'NONE', #10711, #846 ) ;
#1607=ORIENTED_EDGE ( 'NONE', *, *, #8386, .T. ) ;
#1608=LINE ( 'NONE', #7425, #3319 ) ;
#1615=VERTEX_POINT ( 'NONE', #11629 ) ;
#1617=ORIENTED_EDGE ( 'NONE', *, *, #4280, .F. ) ;
#1623=CARTESIAN_POINT ( 'NONE',  ( -379.7747414317349808, 63.03754323421768646, -131.1733032197525119 ) ) ;
#1624=CARTESIAN_POINT ( 'NONE',  ( -59.99999999999998579, 24.00000000000001421, -126.4213562373090696 ) ) ;
#1625=ORIENTED_EDGE ( 'NONE', *, *, #7440, .F. ) ;
#1630=ADVANCED_FACE ( 'NONE', ( #6917 ), #5866, .T. ) ;
#1635=CARTESIAN_POINT ( 'NONE',  ( -384.9998751003590201, 83.30729021256857436, -104.6803604098840168 ) ) ;
#1637=DIRECTION ( 'NONE',  ( 0.000000000000000000, 0.9467162604879117982, -0.3220688158263456113 ) ) ;
#1647=DIRECTION ( 'NONE',  ( 1.000000000000000000, 0.000000000000000000, 0.000000000000000000 ) ) ;
#1649=CARTESIAN_POINT ( 'NONE',  ( -822.1849787629541879, 73.94083650471891644, -142.9856651621327046 ) ) ;
#1652=CARTESIAN_POINT ( 'NONE',  ( -370.0238914150202731, 56.07874637648789928, -129.5483826961032037 ) ) ;
#1660=AXIS2_PLACEMENT_3D ( 'NONE', #172, #6791, #5799 ) ;
#1677=ORIENTED_EDGE ( 'NONE', *, *, #12039, .T. ) ;
#1684=ORIENTED_EDGE ( 'NONE', *, *, #11803, .T. ) ;
#1686=EDGE_CURVE ( 'NONE', #192, #10150, #2698, .T. ) ;
#1688=CARTESIAN_POINT ( 'NONE',  ( -370.1689562966705580, 56.44580195161717029, -131.5601801359200920 ) ) ;
#1689=DIRECTION ( 'NONE',  ( -8.163404592832030268E-17, 1.000000000000000000, -0.000000000000000000 ) ) ;
#1699=LINE ( 'NONE', #7261, #4772 ) ;
#1704=EDGE_CURVE ( 'NONE', #6191, #9127, #4013, .T. ) ;
#1707=CARTESIAN_POINT ( 'NONE',  ( -82.49999999999998579, 152.0000000000000000, -126.4213562373088564 ) ) ;
#1708=VERTEX_POINT ( 'NONE', #11240 ) ;
#1712=ORIENTED_EDGE ( 'NONE', *, *, #6388, .F. ) ;
#1715=AXIS2_PLACEMENT_3D ( 'NONE', #7182, #3409, #3235 ) ;
#1717=CARTESIAN_POINT ( 'NONE',  ( -822.1919554870369211, 73.93830887977112809, -106.3769876045755467 ) ) ;
#1718=CARTESIAN_POINT ( 'NONE',  ( -826.9024563477383936, 74.71743289348825101, -143.3087845970614183 ) ) ;
#1719=ORIENTED_EDGE ( 'NONE', *, *, #8523, .F. ) ;
#1723=CARTESIAN_POINT ( 'NONE',  ( -374.0275851353517851, 95.01260271039970462, -109.3552309949570400 ) ) ;
#1726=EDGE_CURVE ( 'NONE', #5232, #609, #4808, .T. ) ;
#1730=CARTESIAN_POINT ( 'NONE',  ( -22.49999999999999289, 139.9999999999999716, -126.4213562373092685 ) ) ;
#1736=CIRCLE ( 'NONE', #11795, 7.500000000000007994 ) ;
#1744=ORIENTED_EDGE ( 'NONE', *, *, #860, .F. ) ;
#1746=CARTESIAN_POINT ( 'NONE',  ( -374.4050532074698481, 92.42149850801368416, -141.8266576912406833 ) ) ;
#1755=ORIENTED_EDGE ( 'NONE', *, *, #4932, .T. ) ;
#1756=CARTESIAN_POINT ( 'NONE',  ( -374.0178982243409109, 68.97857190266184091, -139.9467288357900827 ) ) ;
#1760=VECTOR ( 'NONE', #8649, 1000.000000000000000 ) ;
#1761=EDGE_CURVE ( 'NONE', #10791, #8166, #4560, .T. ) ;
#1762=CARTESIAN_POINT ( 'NONE',  ( -305.0000000000000568, 139.9999999999999716, -89.68077099980384048 ) ) ;
#1767=CARTESIAN_POINT ( 'NONE',  ( -59.99999999999998579, 12.00000000000001421, -126.4213562373090696 ) ) ;
#1770=ORIENTED_EDGE ( 'NONE', *, *, #2177, .T. ) ;
#1771=CARTESIAN_POINT ( 'NONE',  ( -828.3910170805050939, 80.72627522873268902, -144.6407408995347339 ) ) ;
#1783=CARTESIAN_POINT ( 'NONE',  ( -828.8285638327206470, 78.67432280806529832, -144.4023295390027215 ) ) ;
#1786=CARTESIAN_POINT ( 'NONE',  ( -371.8534480886071378, 61.21526739536749773, -143.1506241535973061 ) ) ;
#1788=ORIENTED_EDGE ( 'NONE', *, *, #5842, .T. ) ;
#1798=CARTESIAN_POINT ( 'NONE',  ( -372.7288769611630528, 100.8944622026212983, -118.0665564160781855 ) ) ;
#1799=EDGE_CURVE ( 'NONE', #9710, #8281, #1442, .T. ) ;
#1802=CYLINDRICAL_SURFACE ( 'NONE', #6617, 7.500000000000007105 ) ;
#1805=CARTESIAN_POINT ( 'NONE',  ( -382.1275881780431973, 96.19125754664578665, -138.8335771761920796 ) ) ;
#1810=VERTEX_POINT ( 'NONE', #5344 ) ;
#1816=CIRCLE ( 'NONE', #8529, 7.500000000000007105 ) ;
#1818=CARTESIAN_POINT ( 'NONE',  ( -381.5707893087703724, 66.54686343221263201, -137.3937270100335866 ) ) ;
#1821=DIRECTION ( 'NONE',  ( -1.000000000000000000, 0.000000000000000000, 0.000000000000000000 ) ) ;
#1830=CARTESIAN_POINT ( 'NONE',  ( -379.5881075290514559, 101.2865363140498403, -130.0868282690590831 ) ) ;
#1832=CARTESIAN_POINT ( 'NONE',  ( -820.4056028115145409, 82.32260517263510735, -144.6785023965173025 ) ) ;
#1834=CARTESIAN_POINT ( 'NONE',  ( -828.8285638327206470, 78.67432280806529832, -104.9592124606049879 ) ) ;
#1849=ORIENTED_EDGE ( 'NONE', *, *, #1121, .T. ) ;
#1855=VERTEX_POINT ( 'NONE', #855 ) ;
#1857=DIRECTION ( 'NONE',  ( -0.000000000000000000, -0.000000000000000000, 1.000000000000000000 ) ) ;
#1860=CARTESIAN_POINT ( 'NONE',  ( -305.0000000000000568, 81.99999999999995737, -89.68077099980384048 ) ) ;
#1865=CARTESIAN_POINT ( 'NONE',  ( -172.5000000000000000, -9.213203435596478030, -126.4213562373082453 ) ) ;
#1867=VECTOR ( 'NONE', #5188, 1000.000000000000000 ) ;
#1880=CARTESIAN_POINT ( 'NONE',  ( -374.3481803600093372, 71.08267651485977012, -141.5671192069848701 ) ) ;
#1881=DIRECTION ( 'NONE',  ( 1.000000000000000000, 0.000000000000000000, 0.000000000000000000 ) ) ;
#1882=CARTESIAN_POINT ( 'NONE',  ( -384.7075901990183411, 77.40006559035658995, -105.2059176660476396 ) ) ;
#1888=CARTESIAN_POINT ( 'NONE',  ( -240.0000000000000000, 151.9999999999999716, -126.4213562373078190 ) ) ;
#1897=CARTESIAN_POINT ( 'NONE',  ( -373.6479907027180616, 95.69918402684290015, -99.08269489361265414 ) ) ;
#1900=LINE ( 'NONE', #3063, #9448 ) ;
#1902=FACE_OUTER_BOUND ( 'NONE', #925, .T. ) ;
#1906=CARTESIAN_POINT ( 'NONE',  ( -374.7132803760889601, 89.60697909709962516, -106.0899807314232248 ) ) ;
#1910=DIRECTION ( 'NONE',  ( -8.163404592832031500E-17, 1.000000000000000000, 0.000000000000000000 ) ) ;
#1913=ORIENTED_EDGE ( 'NONE', *, *, #824, .F. ) ;
#1914=DIRECTION ( 'NONE',  ( -8.163404592832030268E-17, 1.000000000000000000, -0.000000000000000000 ) ) ;
#1916=CARTESIAN_POINT ( 'NONE',  ( -112.4999999999999858, 152.0000000000000000, -126.4213562373086575 ) ) ;
#1920=FACE_OUTER_BOUND ( 'NONE', #183, .T. ) ;
#1924=CARTESIAN_POINT ( 'NONE',  ( -374.6521690518432024, 90.20916286035372877, -142.9852835970012279 ) ) ;
#1931=ORIENTED_EDGE ( 'NONE', *, *, #4795, .T. ) ;
#1935=FACE_OUTER_BOUND ( 'NONE', #4634, .T. ) ;
#1937=STYLED_ITEM ( 'NONE', ( #3274 ), #8029 ) ;
#1938=CARTESIAN_POINT ( 'NONE',  ( -385.0061886013530739, 82.02011007860102154, -144.6917801619403861 ) ) ;
#1940=CARTESIAN_POINT ( 'NONE',  ( -374.7231203874862331, 74.61313258587077257, -106.0425182818924554 ) ) ;
#1942=AXIS2_PLACEMENT_3D ( 'NONE', #4530, #6845, #6192 ) ;
#1953=CARTESIAN_POINT ( 'NONE',  ( -380.0196196571620817, 63.47433729084224296, -117.1214152238070341 ) ) ;
#1956=CARTESIAN_POINT ( 'NONE',  ( -820.9141234758953942, 82.74039896267167649, -144.6672699209827613 ) ) ;
#1957=CARTESIAN_POINT ( 'NONE',  ( -371.8698477746299886, 102.7100032247106469, -106.2096734411371557 ) ) ;
#1959=EDGE_LOOP ( 'NONE', ( #10356, #3461, #11148, #3797, #7547, #7980 ) ) ;
#1968=AXIS2_PLACEMENT_3D ( 'NONE', #7539, #11492, #6671 ) ;
#1969=VERTEX_POINT ( 'NONE', #3753 ) ;
#1971=CARTESIAN_POINT ( 'NONE',  ( -374.2661435795450871, 93.45316928466465356, -108.1938755228533182 ) ) ;
#1974=ORIENTED_EDGE ( 'NONE', *, *, #4514, .T. ) ;
#1984=EDGE_CURVE ( 'NONE', #6153, #6536, #4698, .T. ) ;
#1986=LINE ( 'NONE', #1063, #10737 ) ;
#1988=VERTEX_POINT ( 'NONE', #8472 ) ;
#1990=CARTESIAN_POINT ( 'NONE',  ( 7.500000000000008882, 152.0000000000000000, -126.4213562373094959 ) ) ;
#1994=DIRECTION ( 'NONE',  ( 0.000000000000000000, 0.000000000000000000, 1.000000000000000000 ) ) ;
#1999=CARTESIAN_POINT ( 'NONE',  ( -374.9802614396505760, 80.28172288411161617, -154.6205875143999435 ) ) ;
#2001=CARTESIAN_POINT ( 'NONE',  ( -382.7837046478651928, 69.53043186086833316, -109.0405781650321018 ) ) ;
#2005=ORIENTED_EDGE ( 'NONE', *, *, #3262, .F. ) ;
#2011=CARTESIAN_POINT ( 'NONE',  ( -379.7921418149325063, 63.07164944986214294, -118.2218589047913611 ) ) ;
#2013=ORIENTED_EDGE ( 'NONE', *, *, #6969, .F. ) ;
#2019=DIRECTION ( 'NONE',  ( -8.163404592832030268E-17, 1.000000000000000000, -0.000000000000000000 ) ) ;
#2024=CIRCLE ( 'NONE', #11878, 7.500000000000020428 ) ;
#2026=CARTESIAN_POINT ( 'NONE',  ( 0.000000000000000000, 152.0000000000000000, -89.68077099980384048 ) ) ;
#2027=ORIENTED_EDGE ( 'NONE', *, *, #8509, .F. ) ;
#2029=EDGE_CURVE ( 'NONE', #6191, #2820, #8606, .T. ) ;
#2034=EDGE_LOOP ( 'NONE', ( #2196, #8986 ) ) ;
#2036=CARTESIAN_POINT ( 'NONE',  ( -818.8285638327206470, 78.67432280806531253, -104.9592124606049879 ) ) ;
#2042=VERTEX_POINT ( 'NONE', #2026 ) ;
#2045=CIRCLE ( 'NONE', #10527, 7.500000000000007105 ) ;
#2046=PLANE ( 'NONE',  #629 ) ;
#2047=EDGE_LOOP ( 'NONE', ( #3070, #10949 ) ) ;
#2052=FACE_BOUND ( 'NONE', #6778, .T. ) ;
#2057=CARTESIAN_POINT ( 'NONE',  ( -373.8927214104571135, 69.57595966422515232, -151.1258107129636699 ) ) ;
#2059=CARTESIAN_POINT ( 'NONE',  ( -383.2380640590296252, 70.81816280502410166, -108.0477105264665880 ) ) ;
#2068=DIRECTION ( 'NONE',  ( -1.000000000000000000, 0.000000000000000000, 0.000000000000000000 ) ) ;
#2075=CARTESIAN_POINT ( 'NONE',  ( -384.1464637028664697, 74.21013607762992592, -106.2506866248873365 ) ) ;
#2078=VERTEX_POINT ( 'NONE', #5728 ) ;
#2079=EDGE_CURVE ( 'NONE', #7375, #11612, #2045, .T. ) ;
#2085=DIRECTION ( 'NONE',  ( -8.163404592832030268E-17, 1.000000000000000000, -0.000000000000000000 ) ) ;
#2086=DIRECTION ( 'NONE',  ( -8.163404592832030268E-17, 1.000000000000000000, -0.000000000000000000 ) ) ;
#2087=PRODUCT_DEFINITION_CONTEXT ( 'detailed design', #6531, 'design' ) ;
#2088=VECTOR ( 'NONE', #6452, 1000.000000000000000 ) ;
#2090=DIRECTION ( 'NONE',  ( 0.000000000000000000, 0.000000000000000000, 1.000000000000000000 ) ) ;
#2103=CARTESIAN_POINT ( 'NONE',  ( 1.142876642996484321E-14, 24.00000000000001421, -126.4213562373094959 ) ) ;
#2104=CARTESIAN_POINT ( 'NONE',  ( -150.0000000000000000, -9.213203435596451385, -126.4213562373084301 ) ) ;
#2108=ORIENTED_EDGE ( 'NONE', *, *, #542, .T. ) ;
#2112=ORIENTED_EDGE ( 'NONE', *, *, #1121, .F. ) ;
#2114=ORIENTED_EDGE ( 'NONE', *, *, #414, .F. ) ;
#2115=CARTESIAN_POINT ( 'NONE',  ( -381.8407521777220950, 96.85938717894678973, -138.1176283752880067 ) ) ;
#2119=CARTESIAN_POINT ( 'NONE',  ( -374.9887786383590651, 80.39322394422208617, -144.6212526005259065 ) ) ;
#2121=CARTESIAN_POINT ( 'NONE',  ( -374.9884691243568113, 80.37146653597520185, -104.7419479422377577 ) ) ;
#2123=CARTESIAN_POINT ( 'NONE',  ( -270.0000000000000000, 24.00000000000000711, -126.4213562373076059 ) ) ;
#2130=AXIS2_PLACEMENT_3D ( 'NONE', #11448, #8548, #1136 ) ;
#2133=ORIENTED_EDGE ( 'NONE', *, *, #4354, .T. ) ;
#2135=CARTESIAN_POINT ( 'NONE',  ( -384.9561085268001648, 84.12206627636906831, -104.7580990804535759 ) ) ;
#2142=CYLINDRICAL_SURFACE ( 'NONE', #5804, 7.500000000000007105 ) ;
#2143=VECTOR ( 'NONE', #5403, 1000.000000000000000 ) ;
#2147=CIRCLE ( 'NONE', #9240, 7.500000000000020428 ) ;
#2152=ADVANCED_FACE ( 'NONE', ( #5669 ), #9445, .F. ) ;
#2160=ORIENTED_EDGE ( 'NONE', *, *, #2605, .T. ) ;
#2165=CLOSED_SHELL ( 'NONE', ( #4044, #4135, #1107, #10753, #9538, #7591, #8135, #6025, #5853, #8512, #8603, #6024, #5151, #5797, #10679, #10361, #11136, #7834, #1408, #7906, #4103, #8920, #9107, #11510, #1630, #8821, #4879, #2972, #3912, #10785, #11835, #5452, #478, #9270, #5298, #10516, #22, #2152, #11139, #2444, #6303, #11118, #1277, #5788, #3667, #11622, #5767, #8124, #11426, #2822, #9473, #7376, #11174, #12222, #6697, #7422, #553, #12229, #270 ) ) ;
#2168=CARTESIAN_POINT ( 'NONE',  ( -210.0000000000000000, 151.9999999999999716, -126.4213562373080180 ) ) ;
#2169=CARTESIAN_POINT ( 'NONE',  ( -29.99999999999998934, 24.00000000000001421, -126.4213562373092685 ) ) ;
#2177=EDGE_CURVE ( 'NONE', #10646, #7797, #339, .T. ) ;
#2178=CARTESIAN_POINT ( 'NONE',  ( -380.2702075887810906, 100.0761580381868896, -133.3173879207189998 ) ) ;
#2190=CARTESIAN_POINT ( 'NONE',  ( -202.4999999999999716, 139.9999999999999716, -126.4213562373080180 ) ) ;
#2191=CARTESIAN_POINT ( 'NONE',  ( -380.7160366723977063, 64.77876409789038803, -114.4938704800854907 ) ) ;
#2192=EDGE_LOOP ( 'NONE', ( #1719, #9089 ) ) ;
#2193=CARTESIAN_POINT ( 'NONE',  ( -262.5000000000000000, 151.9999999999999716, -126.4213562373076059 ) ) ;
#2196=ORIENTED_EDGE ( 'NONE', *, *, #4570, .F. ) ;
#2211=AXIS2_PLACEMENT_3D ( 'NONE', #3083, #8829, #4817 ) ;
#2215=EDGE_CURVE ( 'NONE', #8134, #10520, #2245, .T. ) ;
#2216=CARTESIAN_POINT ( 'NONE',  ( -822.6918648528270523, 83.54617135775964698, -104.7406007859484873 ) ) ;
#2220=ORIENTED_EDGE ( 'NONE', *, *, #12118, .F. ) ;
#2221=CARTESIAN_POINT ( 'NONE',  ( -305.0000000000000568, 81.99999999999995737, -89.68077099980384048 ) ) ;
#2222=AXIS2_PLACEMENT_3D ( 'NONE', #11831, #3287, #8906 ) ;
#2227=LINE ( 'NONE', #11634, #3383 ) ;
#2228=ORIENTED_EDGE ( 'NONE', *, *, #9358, .F. ) ;
#2231=EDGE_CURVE ( 'NONE', #10646, #9219, #7977, .T. ) ;
#2236=DIRECTION ( 'NONE',  ( 1.000000000000000000, 0.000000000000000000, 0.000000000000000000 ) ) ;
#2237=DIRECTION ( 'NONE',  ( -1.000000000000000000, 0.000000000000000000, 0.000000000000000000 ) ) ;
#2241=( NAMED_UNIT ( * ) PLANE_ANGLE_UNIT ( ) SI_UNIT ( $, .RADIAN. ) );
#2244=EDGE_LOOP ( 'NONE', ( #4771, #7124 ) ) ;
#2245=CIRCLE ( 'NONE', #4032, 7.500000000000007105 ) ;
#2255=ORIENTED_EDGE ( 'NONE', *, *, #6451, .F. ) ;
#2264=CIRCLE ( 'NONE', #11341, 10.00000000000000355 ) ;
#2265=ORIENTED_EDGE ( 'NONE', *, *, #7747, .F. ) ;
#2266=CIRCLE ( 'NONE', #1464, 7.500000000000007105 ) ;
#2272=DIRECTION ( 'NONE',  ( 0.000000000000000000, 1.000000000000000000, -0.000000000000000000 ) ) ;
#2276=CYLINDRICAL_SURFACE ( 'NONE', #8493, 7.500000000000007105 ) ;
#2281=FACE_BOUND ( 'NONE', #9539, .T. ) ;
#2283=CYLINDRICAL_SURFACE ( 'NONE', #12150, 7.500000000000007105 ) ;
#2284=DIRECTION ( 'NONE',  ( -1.000000000000000000, 0.000000000000000000, 0.000000000000000000 ) ) ;
#2285=EDGE_CURVE ( 'NONE', #5774, #192, #3821, .T. ) ;
#2295=CARTESIAN_POINT ( 'NONE',  ( -380.3383793650497751, 64.05796225469710237, -115.8204086816914611 ) ) ;
#2303=VECTOR ( 'NONE', #12, 1000.000000000000000 ) ;
#2304=ORIENTED_EDGE ( 'NONE', *, *, #11586, .T. ) ;
#2305=ORIENTED_EDGE ( 'NONE', *, *, #4849, .F. ) ;
#2316=DIRECTION ( 'NONE',  ( -8.163404592832030268E-17, 1.000000000000000000, -0.000000000000000000 ) ) ;
#2317=EDGE_CURVE ( 'NONE', #9984, #5834, #5992, .T. ) ;
#2318=AXIS2_PLACEMENT_3D ( 'NONE', #9709, #1132, #11503 ) ;
#2319=EDGE_CURVE ( 'NONE', #11283, #4655, #4613, .T. ) ;
#2320=CARTESIAN_POINT ( 'NONE',  ( -210.0000000000000000, 139.9999999999999716, -126.4213562373080180 ) ) ;
#2321=DIRECTION ( 'NONE',  ( 0.000000000000000000, 1.000000000000000000, -0.000000000000000000 ) ) ;
#2324=DIRECTION ( 'NONE',  ( -8.163404592832030268E-17, 1.000000000000000000, -0.000000000000000000 ) ) ;
#2327=CIRCLE ( 'NONE', #8836, 7.500000000000007105 ) ;
#2333=CARTESIAN_POINT ( 'NONE',  ( -142.5000000000000000, -9.213203435596451385, -126.4213562373084301 ) ) ;
#2339=DIRECTION ( 'NONE',  ( -1.000000000000000000, 0.000000000000000000, 0.000000000000000000 ) ) ;
#2342=CARTESIAN_POINT ( 'NONE',  ( -370.6747336736685838, 106.2267788995130786, -113.0893085367774376 ) ) ;
#2352=CYLINDRICAL_SURFACE ( 'NONE', #3013, 57.99999999999999289 ) ;
#2355=EDGE_LOOP ( 'NONE', ( #11164, #6242, #4884, #6676 ) ) ;
#2356=DIRECTION ( 'NONE',  ( -1.000000000000000000, 0.000000000000000000, 0.000000000000000000 ) ) ;
#2357=CARTESIAN_POINT ( 'NONE',  ( -382.0060323104738700, 67.53962357491931812, -138.5094348483520150 ) ) ;
#2359=CYLINDRICAL_SURFACE ( 'NONE', #10041, 7.500000000000007994 ) ;
#2364=ORIENTED_EDGE ( 'NONE', *, *, #6921, .T. ) ;
#2371=CARTESIAN_POINT ( 'NONE',  ( -379.6770763389447438, 101.1299400358934690, -118.8159555003075809 ) ) ;
#2374=EDGE_CURVE ( 'NONE', #9074, #6366, #4813, .T. ) ;
#2375=DIRECTION ( 'NONE',  ( -8.163404592832030268E-17, 1.000000000000000000, -0.000000000000000000 ) ) ;
#2391=CARTESIAN_POINT ( 'NONE',  ( -828.5765974139357013, 80.27527354417595973, -104.7529721962248601 ) ) ;
#2393=EDGE_CURVE ( 'NONE', #10150, #7370, #11724, .T. ) ;
#2400=CARTESIAN_POINT ( 'NONE',  ( -374.4047048906529653, 72.86532638985215726, -96.54417189472898997 ) ) ;
#2401=CIRCLE ( 'NONE', #11871, 7.500000000000007105 ) ;
#2406=CARTESIAN_POINT ( 'NONE',  ( -380.4123712287169496, 64.19693960509795261, -133.8127555985722381 ) ) ;
#2409=CARTESIAN_POINT ( 'NONE',  ( -373.6838828167635711, 95.52325971351345402, -150.4055153106844216 ) ) ;
#2410=LINE ( 'NONE', #1491, #7985 ) ;
#2421=CARTESIAN_POINT ( 'NONE',  ( -379.4946887727529656, 101.4434214888139820, -119.9580570101217916 ) ) ;
#2423=ORIENTED_EDGE ( 'NONE', *, *, #121, .F. ) ;
#2428=VECTOR ( 'NONE', #10558, 1000.000000000000000 ) ;
#2432=PLANE ( 'NONE',  #1018 ) ;
#2433=CARTESIAN_POINT ( 'NONE',  ( -374.7331952787391174, 88.13045056185990234, -95.50322499346698635 ) ) ;
#2434=ORIENTED_EDGE ( 'NONE', *, *, #12039, .F. ) ;
#2435=DIRECTION ( 'NONE',  ( 2.040851148208007875E-17, -1.000000000000000000, -0.000000000000000000 ) ) ;
#2438=CIRCLE ( 'NONE', #2645, 7.500000000000007105 ) ;
#2444=ADVANCED_FACE ( 'NONE', ( #9574 ), #8710, .F. ) ;
#2448=AXIS2_PLACEMENT_3D ( 'NONE', #7157, #1531, #728 ) ;
#2466=ORIENTED_EDGE ( 'NONE', *, *, #4354, .F. ) ;
#2473=CARTESIAN_POINT ( 'NONE',  ( -232.4999999999999716, 151.9999999999999716, -126.4213562373078190 ) ) ;
#2476=CARTESIAN_POINT ( 'NONE',  ( -89.99999999999998579, -9.213203435596451385, -126.4213562373088564 ) ) ;
#2485=CARTESIAN_POINT ( 'NONE',  ( -370.2343257278625970, 56.60651921569737510, -116.8345502163405030 ) ) ;
#2486=CARTESIAN_POINT ( 'NONE',  ( -379.7826593342579713, 100.9462791126746595, -118.2474210935536973 ) ) ;
#2497=CARTESIAN_POINT ( 'NONE',  ( -375.0052866622255010, 81.99894079391765445, -104.6528133239954457 ) ) ;
#2510=CIRCLE ( 'NONE', #10419, 7.500000000000007105 ) ;
#2515=DIRECTION ( 'NONE',  ( 1.000000000000000000, 0.000000000000000000, 0.000000000000000000 ) ) ;
#2520=AXIS2_PLACEMENT_3D ( 'NONE', #11776, #7413, #805 ) ;
#2522=ORIENTED_EDGE ( 'NONE', *, *, #8570, .T. ) ;
#2526=CARTESIAN_POINT ( 'NONE',  ( -247.5000000000000000, -9.213203435596478030, -126.4213562373078190 ) ) ;
#2534=CARTESIAN_POINT ( 'NONE',  ( -379.1619848709566440, 102.0000000000000142, -124.6807709998038405 ) ) ;
#2541=ORIENTED_EDGE ( 'NONE', *, *, #5149, .F. ) ;
#2544=ORIENTED_EDGE ( 'NONE', *, *, #824, .T. ) ;
#2547=CARTESIAN_POINT ( 'NONE',  ( -372.4042090581564253, 61.94512028621924316, -124.6876203640234451 ) ) ;
#2563=EDGE_LOOP ( 'NONE', ( #2112, #7915, #6425, #11031 ) ) ;
#2568=CARTESIAN_POINT ( 'NONE',  ( -30.00000000000000000, 152.0000000000000000, -126.4213562373092685 ) ) ;
#2571=CARTESIAN_POINT ( 'NONE',  ( -828.8205192778966648, 78.34647195564905076, -144.3449412327537686 ) ) ;
#2575=ORIENTED_EDGE ( 'NONE', *, *, #6553, .T. ) ;
#2589=CARTESIAN_POINT ( 'NONE',  ( -379.2139264233433664, 101.9143973957450271, -126.6420371101448552 ) ) ;
#2594=VERTEX_POINT ( 'NONE', #1295 ) ;
#2602=VERTEX_POINT ( 'NONE', #1467 ) ;
#2605=EDGE_CURVE ( 'NONE', #10791, #818, #5424, .T. ) ;
#2607=CARTESIAN_POINT ( 'NONE',  ( -371.2164454780093479, 59.29687532392634353, -139.7481348488436765 ) ) ;
#2610=EDGE_CURVE ( 'NONE', #4244, #11206, #8395, .T. ) ;
#2621=CARTESIAN_POINT ( 'NONE',  ( -822.2160636604378396, 83.41847921025862433, -144.6308011508168079 ) ) ;
#2630=CARTESIAN_POINT ( 'NONE',  ( -824.9897882054046931, 73.80822682502996201, -106.4353286633422471 ) ) ;
#2640=ADVANCED_BREP_SHAPE_REPRESENTATION ( '', ( #8029, #11957 ), #4670 ) ;
#2642=DIRECTION ( 'NONE',  ( -0.000000000000000000, -1.000000000000000000, -0.000000000000000000 ) ) ;
#2643=CARTESIAN_POINT ( 'NONE',  ( -371.9152332062730579, 61.43342894527527420, -105.9795901510680096 ) ) ;
#2645=AXIS2_PLACEMENT_3D ( 'NONE', #2657, #9081, #4652 ) ;
#2646=AXIS2_PLACEMENT_3D ( 'NONE', #3933, #4973, #9496 ) ;
#2650=DIRECTION ( 'NONE',  ( -1.000000000000000000, 0.000000000000000000, 0.000000000000000000 ) ) ;
#2651=CARTESIAN_POINT ( 'NONE',  ( -305.0000000000000568, 151.9999999999999716, -89.68077099980384048 ) ) ;
#2655=CIRCLE ( 'NONE', #9167, 7.500000000000007105 ) ;
#2657=CARTESIAN_POINT ( 'NONE',  ( -29.99999999999998579, 12.00000000000001776, -126.4213562373092685 ) ) ;
#2668=VECTOR ( 'NONE', #4589, 1000.000000000000000 ) ;
#2671=CARTESIAN_POINT ( 'NONE',  ( -67.49999999999998579, -9.213203435596451385, -126.4213562373090696 ) ) ;
#2672=ORIENTED_EDGE ( 'NONE', *, *, #4894, .T. ) ;
#2673=CARTESIAN_POINT ( 'NONE',  ( -373.9743428662257543, 68.72570060467459996, -139.7265316089925022 ) ) ;
#2675=EDGE_CURVE ( 'NONE', #2042, #4719, #5008, .T. ) ;
#2688=CARTESIAN_POINT ( 'NONE',  ( -826.8836092318784949, 82.64591421739807231, -144.6711677827315157 ) ) ;
#2692=ORIENTED_EDGE ( 'NONE', *, *, #9999, .T. ) ;
#2698=LINE ( 'NONE', #12100, #10329 ) ;
#2701=FACE_OUTER_BOUND ( 'NONE', #2563, .T. ) ;
#2703=CARTESIAN_POINT ( 'NONE',  ( -827.6116022231220768, 75.38889084172069488, -143.5581011396505744 ) ) ;
#2707=CARTESIAN_POINT ( 'NONE',  ( -373.6129858352072119, 95.87061353962586452, -99.20626003773914192 ) ) ;
#2716=CIRCLE ( 'NONE', #6468, 7.500000000000007105 ) ;
#2728=CARTESIAN_POINT ( 'NONE',  ( -247.5000000000000000, 12.00000000000001066, -126.4213562373078190 ) ) ;
#2729=CARTESIAN_POINT ( 'NONE',  ( -373.8878671940757386, 94.45254164238392036, -151.1084388673575063 ) ) ;
#2734=AXIS2_PLACEMENT_3D ( 'NONE', #7147, #10795, #3307 ) ;
#2741=CARTESIAN_POINT ( 'NONE',  ( -371.0707588476642513, 58.87632496566943985, -138.8882774118476107 ) ) ;
#2756=CARTESIAN_POINT ( 'NONE',  ( -379.2183536796136991, 101.9077751251720372, -126.8862509569658670 ) ) ;
#2759=CARTESIAN_POINT ( 'NONE',  ( -825.4446906002082187, 83.41738352290668956, -144.6308861023091197 ) ) ;
#2768=FACE_OUTER_BOUND ( 'NONE', #666, .T. ) ;
#2769=CARTESIAN_POINT ( 'NONE',  ( -825.6238610960850792, 74.00482032089485074, -106.3482309385107243 ) ) ;
#2772=EDGE_CURVE ( 'NONE', #1708, #4712, #6773, .T. ) ;
#2773=EDGE_LOOP ( 'NONE', ( #1327, #5628, #9622, #9159 ) ) ;
#2774=CARTESIAN_POINT ( 'NONE',  ( -373.9906543607759772, 70.14504041414527080, -151.4544406809787347 ) ) ;
#2775=CARTESIAN_POINT ( 'NONE',  ( -383.4148409544956166, 92.56808650636575919, -107.6977636917801533 ) ) ;
#2781=ORIENTED_EDGE ( 'NONE', *, *, #7595, .T. ) ;
#2789=EDGE_LOOP ( 'NONE', ( #5495, #7082 ) ) ;
#2791=CARTESIAN_POINT ( 'NONE',  ( -383.0516306480785147, 93.70208505889323192, -140.9032205339583754 ) ) ;
#2800=FACE_BOUND ( 'NONE', #250, .T. ) ;
#2801=CARTESIAN_POINT ( 'NONE',  ( -384.2952596656363085, 74.92966664680659505, -143.3922324125414320 ) ) ;
#2803=CARTESIAN_POINT ( 'NONE',  ( -384.5205618194315207, 76.13527207948695263, -105.5487487501123383 ) ) ;
#2805=ORIENTED_EDGE ( 'NONE', *, *, #8944, .F. ) ;
#2806=B_SPLINE_CURVE_WITH_KNOTS ( 'NONE', 3,
 ( #6647, #3604, #3866, #970, #8400, #2819, #7395, #784, #10415, #10238, #5597, #11167, #5534, #9308, #851, #1032, #9374, #10480, #1957, #6707, #4620, #4797, #917, #6587, #10355, #1897, #5660, #4741, #24, #5100, #9576, #2433, #8012, #9045, #514, #7136, #8655, #10901 ),
 .UNSPECIFIED., .F., .F.,
 ( 4, 2, 2, 2, 2, 2, 2, 2, 2, 2, 2, 2, 2, 2, 2, 2, 2, 2, 4 ),
 ( 0.1699018821680253755, 0.1767590822639642234, 0.1784733822879489284, 0.1801876823119336335, 0.1836162823599029603, 0.1870448824078722594, 0.1887591824318569367, 0.1904734824558415862, 0.1973306825517801288, 0.2007592825997494279, 0.2041878826477186992, 0.2076164826956879983, 0.2093307827196726478, 0.2110450827436572974, 0.2144736827916266242, 0.2179022828395959510, 0.2196165828635806005, 0.2213308828875652778, 0.2247594829355346324 ),
 .UNSPECIFIED. ) ;
#2810=CIRCLE ( 'NONE', #9719, 7.500000000000007105 ) ;
#2819=CARTESIAN_POINT ( 'NONE',  ( -369.8931053733606404, 108.2466269641216456, -125.4256155901781256 ) ) ;
#2820=VERTEX_POINT ( 'NONE', #2828 ) ;
#2822=ADVANCED_FACE ( 'NONE', ( #1902 ), #9442, .F. ) ;
#2823=DIRECTION ( 'NONE',  ( -8.163404592832030268E-17, 1.000000000000000000, -0.000000000000000000 ) ) ;
#2827=FACE_OUTER_BOUND ( 'NONE', #7106, .T. ) ;
#2828=CARTESIAN_POINT ( 'NONE',  ( -375.0000000000000568, 81.99999999999994316, -154.6807709998039115 ) ) ;
#2832=CARTESIAN_POINT ( 'NONE',  ( -372.5030970542207456, 100.5759890823530469, -103.3955147509480810 ) ) ;
#2834=ORIENTED_EDGE ( 'NONE', *, *, #6462, .T. ) ;
#2848=DIRECTION ( 'NONE',  ( -0.000000000000000000, -0.000000000000000000, -1.000000000000000000 ) ) ;
#2853=CIRCLE ( 'NONE', #9748, 7.500000000000007105 ) ;
#2854=CARTESIAN_POINT ( 'NONE',  ( -381.0073242568000182, 98.64321884196588996, -135.7905410542184654 ) ) ;
#2856=ORIENTED_EDGE ( 'NONE', *, *, #1704, .F. ) ;
#2859=EDGE_CURVE ( 'NONE', #2594, #6370, #9222, .T. ) ;
#2861=EDGE_LOOP ( 'NONE', ( #3338, #8774 ) ) ;
#2866=DIRECTION ( 'NONE',  ( 0.000000000000000000, 1.000000000000000000, -0.000000000000000000 ) ) ;
#2869=EDGE_LOOP ( 'NONE', ( #7671, #3456 ) ) ;
#2870=CARTESIAN_POINT ( 'NONE',  ( -384.9074499709351471, 84.64590227528201183, -144.5159070364964577 ) ) ;
#2872=CARTESIAN_POINT ( 'NONE',  ( -374.9921165712652282, 80.64358310894998283, -104.7226567718598034 ) ) ;
#2881=CARTESIAN_POINT ( 'NONE',  ( -383.6153819378109802, 72.10737431220874782, -107.2890747853481912 ) ) ;
#2883=CARTESIAN_POINT ( 'NONE',  ( -820.7807412222807670, 82.64141399635636276, -144.6707558958800917 ) ) ;
#2887=ORIENTED_EDGE ( 'NONE', *, *, #3520, .F. ) ;
#2888=DIRECTION ( 'NONE',  ( -8.163404592832030268E-17, 1.000000000000000000, -0.000000000000000000 ) ) ;
#2890=DIRECTION ( 'NONE',  ( -0.000000000000000000, -0.000000000000000000, -1.000000000000000000 ) ) ;
#2896=CARTESIAN_POINT ( 'NONE',  ( -372.9914527493190235, 98.66121915142865362, -101.4780570701677931 ) ) ;
#2897=ORIENTED_EDGE ( 'NONE', *, *, #1761, .F. ) ;
#2902=DIRECTION ( 'NONE',  ( -0.000000000000000000, -0.000000000000000000, -1.000000000000000000 ) ) ;
#2905=ORIENTED_EDGE ( 'NONE', *, *, #1418, .F. ) ;
#2909=DIRECTION ( 'NONE',  ( 0.000000000000000000, 1.000000000000000000, -0.000000000000000000 ) ) ;
#2915=CARTESIAN_POINT ( 'NONE',  ( -374.7961310093019165, 88.54001489493019506, -143.6624644214829516 ) ) ;
#2926=( GEOMETRIC_REPRESENTATION_CONTEXT ( 3 ) GLOBAL_UNCERTAINTY_ASSIGNED_CONTEXT ( ( #1276 ) ) GLOBAL_UNIT_ASSIGNED_CONTEXT ( ( #10584, #2241, #5947 ) ) REPRESENTATION_CONTEXT ( 'NONE', 'WORKASPACE' ) );
#2928=CARTESIAN_POINT ( 'NONE',  ( -374.9190187245793595, 85.47274673630769826, -154.4334750548730710 ) ) ;
#2930=CARTESIAN_POINT ( 'NONE',  ( -374.8064248916637666, 75.73032293803038328, -105.6470633775803520 ) ) ;
#2934=ORIENTED_EDGE ( 'NONE', *, *, #6014, .F. ) ;
#2938=EDGE_LOOP ( 'NONE', ( #10127, #2672 ) ) ;
#2941=CARTESIAN_POINT ( 'NONE',  ( -240.0000000000000000, -9.213203435596478030, -126.4213562373078190 ) ) ;
#2950=CIRCLE ( 'NONE', #976, 7.500000000000007105 ) ;
#2955=AXIS2_PLACEMENT_3D ( 'NONE', #1294, #7153, #5046 ) ;
#2961=ORIENTED_EDGE ( 'NONE', *, *, #708, .F. ) ;
#2963=DIRECTION ( 'NONE',  ( -8.163404592832030268E-17, 1.000000000000000000, -0.000000000000000000 ) ) ;
#2967=CARTESIAN_POINT ( 'NONE',  ( -187.5000000000000000, -9.213203435596478030, -126.4213562373082453 ) ) ;
#2972=ADVANCED_FACE ( 'NONE', ( #5999, #5064, #128, #9769, #370, #1250, #7801, #5753, #308, #8608, #6805 ), #5874, .F. ) ;
#2977=DIRECTION ( 'NONE',  ( -0.000000000000000000, -0.000000000000000000, -1.000000000000000000 ) ) ;
#2982=CARTESIAN_POINT ( 'NONE',  ( -374.9361197308762712, 78.97941656547077116, -154.4856030161737408 ) ) ;
#2984=CARTESIAN_POINT ( 'NONE',  ( -374.9529056390816208, 78.74775624118257156, -104.9266946745538149 ) ) ;
#2987=ORIENTED_EDGE ( 'NONE', *, *, #8338, .T. ) ;
#2991=EDGE_CURVE ( 'NONE', #1810, #864, #4844, .T. ) ;
#2995=LINE ( 'NONE', #3794, #4830 ) ;
#2997=VERTEX_POINT ( 'NONE', #8953 ) ;
#2998=CARTESIAN_POINT ( 'NONE',  ( -382.1835803329706209, 67.94417042495855696, -110.4054994893419916 ) ) ;
#3004=AXIS2_PLACEMENT_3D ( 'NONE', #8878, #7964, #7026 ) ;
#3012=CARTESIAN_POINT ( 'NONE',  ( -818.8614508132078527, 78.01542073698732338, -105.0789755614316761 ) ) ;
#3013=AXIS2_PLACEMENT_3D ( 'NONE', #7920, #11806, #10752 ) ;
#3016=CARTESIAN_POINT ( 'NONE',  ( -384.6663941904715784, 86.87630725089890404, -105.2815105480247411 ) ) ;
#3022=VERTEX_POINT ( 'NONE', #5361 ) ;
#3026=LINE ( 'NONE', #5624, #10749 ) ;
#3027=CARTESIAN_POINT ( 'NONE',  ( -240.0000000000000000, 139.9999999999999716, -126.4213562373078190 ) ) ;
#3035=CARTESIAN_POINT ( 'NONE',  ( -383.3143487999271883, 92.90250092716235031, -141.4580426032642890 ) ) ;
#3039=CARTESIAN_POINT ( 'NONE',  ( -374.8641704781214230, 87.44069632558799299, -143.9908328712743071 ) ) ;
#3040=CARTESIAN_POINT ( 'NONE',  ( -247.5000000000000000, 151.9999999999999716, -126.4213562373078190 ) ) ;
#3041=CARTESIAN_POINT ( 'NONE',  ( -374.8592969718704353, 76.56519391583682932, -105.3927423586616499 ) ) ;
#3052=CARTESIAN_POINT ( 'NONE',  ( -363.0000000000000568, 81.99999999999995737, -159.6807709998038547 ) ) ;
#3055=CARTESIAN_POINT ( 'NONE',  ( -384.9712557181327952, 80.53912230241294878, -104.7319216108211037 ) ) ;
#3057=ORIENTED_EDGE ( 'NONE', *, *, #165, .T. ) ;
#3058=CIRCLE ( 'NONE', #905, 7.500000000000007105 ) ;
#3063=CARTESIAN_POINT ( 'NONE',  ( -52.49999999999997868, -9.213203435596451385, -126.4213562373090696 ) ) ;
#3064=CARTESIAN_POINT ( 'NONE',  ( -277.5000000000000000, 24.00000000000000711, -126.4213562373076059 ) ) ;
#3067=AXIS2_PLACEMENT_3D ( 'NONE', #2169, #8937, #6051 ) ;
#3070=ORIENTED_EDGE ( 'NONE', *, *, #11211, .F. ) ;
#3071=DIRECTION ( 'NONE',  ( 0.000000000000000000, 0.000000000000000000, 1.000000000000000000 ) ) ;
#3075=VERTEX_POINT ( 'NONE', #11927 ) ;
#3076=CARTESIAN_POINT ( 'NONE',  ( -262.5000000000000000, 12.00000000000001066, -126.4213562373076059 ) ) ;
#3077=EDGE_CURVE ( 'NONE', #10083, #6258, #10939, .T. ) ;
#3081=ORIENTED_EDGE ( 'NONE', *, *, #86, .T. ) ;
#3083=CARTESIAN_POINT ( 'NONE',  ( -150.0000000000000000, 152.0000000000000000, -126.4213562373084301 ) ) ;
#3087=EDGE_CURVE ( 'NONE', #8251, #2602, #5500, .T. ) ;
#3090=( LENGTH_UNIT ( ) NAMED_UNIT ( * ) SI_UNIT ( .MILLI., .METRE. ) );
#3091=ORIENTED_EDGE ( 'NONE', *, *, #10450, .T. ) ;
#3098=AXIS2_PLACEMENT_3D ( 'NONE', #11073, #10143, #5436 ) ;
#3100=CARTESIAN_POINT ( 'NONE',  ( -384.3668374026304946, 88.71950051914814139, -143.5273393398276198 ) ) ;
#3106=ORIENTED_EDGE ( 'NONE', *, *, #8707, .T. ) ;
#3110=CARTESIAN_POINT ( 'NONE',  ( -382.8339495845497709, 94.33502485403373328, -108.9270999018330173 ) ) ;
#3111=EDGE_LOOP ( 'NONE', ( #1511, #11316, #1532, #10987 ) ) ;
#3113=ORIENTED_EDGE ( 'NONE', *, *, #7922, .F. ) ;
#3117=AXIS2_PLACEMENT_3D ( 'NONE', #11424, #6484, #5490 ) ;
#3124=CARTESIAN_POINT ( 'NONE',  ( -240.0000000000000000, 12.00000000000001066, -126.4213562373078190 ) ) ;
#3128=ORIENTED_EDGE ( 'NONE', *, *, #9702, .F. ) ;
#3130=AXIS2_PLACEMENT_3D ( 'NONE', #6989, #1313, #6186 ) ;
#3156=VERTEX_POINT ( 'NONE', #11062 ) ;
#3157=DIRECTION ( 'NONE',  ( 8.163404592832031500E-17, -1.000000000000000000, 0.000000000000000000 ) ) ;
#3159=CARTESIAN_POINT ( 'NONE',  ( -374.6390623088777829, 89.10776330631169628, -153.5629775697134392 ) ) ;
#3160=DIRECTION ( 'NONE',  ( 2.040851148208007875E-17, -1.000000000000000000, -0.000000000000000000 ) ) ;
#3161=CARTESIAN_POINT ( 'NONE',  ( -370.9210819444880940, 58.45107545929887749, -111.3902275226565024 ) ) ;
#3165=ORIENTED_EDGE ( 'NONE', *, *, #3593, .F. ) ;
#3170=CARTESIAN_POINT ( 'NONE',  ( -369.8915433453782953, 55.74834749765059172, -122.7099038825884065 ) ) ;
#3171=FACE_OUTER_BOUND ( 'NONE', #7700, .T. ) ;
#3174=VECTOR ( 'NONE', #8869, 1000.000000000000000 ) ;
#3177=CYLINDRICAL_SURFACE ( 'NONE', #2646, 7.500000000000007105 ) ;
#3195=CARTESIAN_POINT ( 'NONE',  ( -828.8208027856991293, 78.99693817035492316, -104.9068376039972321 ) ) ;
#3208=CARTESIAN_POINT ( 'NONE',  ( -379.4971532347070706, 62.56077224799714998, -129.4206578983209113 ) ) ;
#3210=CARTESIAN_POINT ( 'NONE',  ( -374.3221583053840504, 91.81152812351068349, -152.5535231342899749 ) ) ;
#3214=AXIS2_PLACEMENT_3D ( 'NONE', #719, #12168, #7335 ) ;
#3225=CARTESIAN_POINT ( 'NONE',  ( -380.1314642070832406, 100.3266783612533288, -116.5856617868500962 ) ) ;
#3229=ORIENTED_EDGE ( 'NONE', *, *, #1166, .T. ) ;
#3233=CARTESIAN_POINT ( 'NONE',  ( -127.4999999999999716, -9.213203435596451385, -126.4213562373086575 ) ) ;
#3235=DIRECTION ( 'NONE',  ( -1.000000000000000000, 0.000000000000000000, 0.000000000000000000 ) ) ;
#3238=CIRCLE ( 'NONE', #2448, 35.00000000000000711 ) ;
#3246=LINE ( 'NONE', #2333, #11941 ) ;
#3251=DIRECTION ( 'NONE',  ( 1.000000000000000000, 1.486905836551548832E-16, -0.000000000000000000 ) ) ;
#3256=FACE_BOUND ( 'NONE', #9685, .T. ) ;
#3262=EDGE_CURVE ( 'NONE', #233, #9732, #876, .T. ) ;
#3263=FACE_OUTER_BOUND ( 'NONE', #6900, .T. ) ;
#3274=PRESENTATION_STYLE_ASSIGNMENT (( #11577 ) ) ;
#3281=CARTESIAN_POINT ( 'NONE',  ( -210.0000000000000000, 139.9999999999999716, -126.4213562373080180 ) ) ;
#3287=DIRECTION ( 'NONE',  ( 0.000000000000000000, 1.000000000000000000, -0.000000000000000000 ) ) ;
#3288=VERTEX_POINT ( 'NONE', #9398 ) ;
#3301=ORIENTED_EDGE ( 'NONE', *, *, #6516, .F. ) ;
#3302=AXIS2_PLACEMENT_3D ( 'NONE', #9, #11275, #8614 ) ;
#3307=DIRECTION ( 'NONE',  ( -1.000000000000000000, 0.000000000000000000, 0.000000000000000000 ) ) ;
#3312=CARTESIAN_POINT ( 'NONE',  ( -826.8820017808986904, 82.64709913614485970, -104.6904163631600824 ) ) ;
#3313=CARTESIAN_POINT ( 'NONE',  ( -379.1619848709567009, 61.99999999999992184, -124.1323191136051776 ) ) ;
#3319=VECTOR ( 'NONE', #620, 1000.000000000000000 ) ;
#3327=CARTESIAN_POINT ( 'NONE',  ( -381.0129949838454877, 65.36129575118090429, -135.8392840662656056 ) ) ;
#3331=CARTESIAN_POINT ( 'NONE',  ( -371.1973815542190778, 104.7660296280457715, -139.6871427982646026 ) ) ;
#3336=AXIS2_PLACEMENT_3D ( 'NONE', #7880, #10773, #9848 ) ;
#3338=ORIENTED_EDGE ( 'NONE', *, *, #6229, .T. ) ;
#3340=ORIENTED_EDGE ( 'NONE', *, *, #120, .T. ) ;
#3341=ORIENTED_EDGE ( 'NONE', *, *, #6226, .F. ) ;
#3344=VERTEX_POINT ( 'NONE', #9633 ) ;
#3355=CARTESIAN_POINT ( 'NONE',  ( -374.9690483538964259, 84.66840056888385391, -104.8435496553661181 ) ) ;
#3358=DIRECTION ( 'NONE',  ( -1.000000000000000000, 0.000000000000000000, 0.000000000000000000 ) ) ;
#3377=CARTESIAN_POINT ( 'NONE',  ( -925.0000000000000000, 81.99999999999988631, -124.6807709998038405 ) ) ;
#3382=CARTESIAN_POINT ( 'NONE',  ( -379.3681879713551552, 101.6576152188101503, -128.5919495273215603 ) ) ;
#3383=VECTOR ( 'NONE', #4203, 1000.000000000000000 ) ;
#3385=CARTESIAN_POINT ( 'NONE',  ( -119.9999999999999858, -9.213203435596451385, -126.4213562373086575 ) ) ;
#3386=CARTESIAN_POINT ( 'NONE',  ( 7.500000000000009770, 139.9999999999999716, -126.4213562373094959 ) ) ;
#3391=CIRCLE ( 'NONE', #859, 7.500000000000007105 ) ;
#3397=CARTESIAN_POINT ( 'NONE',  ( -380.8566067580512708, 98.94424270813378541, -114.0399298516432225 ) ) ;
#3401=FACE_OUTER_BOUND ( 'NONE', #4385, .T. ) ;
#3409=DIRECTION ( 'NONE',  ( -8.163404592832031500E-17, 1.000000000000000000, 0.000000000000000000 ) ) ;
#3411=CARTESIAN_POINT ( 'NONE',  ( -375.0005549305242312, 83.05317239051150580, -104.6789509088160628 ) ) ;
#3416=AXIS2_PLACEMENT_3D ( 'NONE', #6745, #10582, #8731 ) ;
#3422=B_SPLINE_CURVE_WITH_KNOTS ( 'NONE', 3,
 ( #9822, #10810, #6121, #364, #6980, #7103, #1362, #2400, #4201, #7040, #1421, #1479, #4023, #7348, #11121, #8224, #11861, #4448, #2643, #11984, #6422, #5722, #7414, #5420, #1537, #5295 ),
 .UNSPECIFIED., .F., .F.,
 ( 4, 2, 2, 2, 2, 2, 2, 2, 2, 2, 2, 2, 4 ),
 ( 0.04496985353261317292, 0.04715854719908585402, 0.04934724086555854206, 0.05372462819850394589, 0.05591332186497667556, 0.05810201553144939135, 0.06247940286439480212, 0.06466809653086749710, 0.06685679019734019901, 0.07123417753028561672, 0.07342287119675831863, 0.07561156486323100667, 0.07998895219617635499 ),
 .UNSPECIFIED. ) ;
#3429=CARTESIAN_POINT ( 'NONE',  ( 0.000000000000000000, 152.0000000000000000, -124.6807709998038405 ) ) ;
#3431=CARTESIAN_POINT ( 'NONE',  ( -823.5000624989246489, 83.67424195610568916, -104.7509713550764872 ) ) ;
#3450=CARTESIAN_POINT ( 'NONE',  ( -305.0000000000000568, 81.99999999999995737, -159.6807709998038547 ) ) ;
#3452=FACE_OUTER_BOUND ( 'NONE', #11635, .T. ) ;
#3456=ORIENTED_EDGE ( 'NONE', *, *, #6780, .F. ) ;
#3459=ORIENTED_EDGE ( 'NONE', *, *, #10530, .T. ) ;
#3461=ORIENTED_EDGE ( 'NONE', *, *, #1704, .T. ) ;
#3462=CARTESIAN_POINT ( 'NONE',  ( -371.2910448380831099, 59.51545945449562680, -140.1702109638846423 ) ) ;
#3468=VERTEX_POINT ( 'NONE', #8590 ) ;
#3486=VECTOR ( 'NONE', #2324, 1000.000000000000000 ) ;
#3487=CARTESIAN_POINT ( 'NONE',  ( -180.0000000000000000, 139.9999999999999716, -126.4213562373082453 ) ) ;
#3489=DIRECTION ( 'NONE',  ( -0.000000000000000000, -0.000000000000000000, 1.000000000000000000 ) ) ;
#3490=CARTESIAN_POINT ( 'NONE',  ( -828.7963533401342602, 78.01901522663797550, -105.0781937692939607 ) ) ;
#3492=CARTESIAN_POINT ( 'NONE',  ( -150.0000000000000000, 12.00000000000001421, -126.4213562373084301 ) ) ;
#3494=CARTESIAN_POINT ( 'NONE',  ( -370.2179477426083167, 56.57026616554610854, -117.1538732267712959 ) ) ;
#3503=VERTEX_POINT ( 'NONE', #7969 ) ;
#3504=ORIENTED_EDGE ( 'NONE', *, *, #5365, .T. ) ;
#3511=CARTESIAN_POINT ( 'NONE',  ( -232.4999999999999716, 139.9999999999999716, -126.4213562373078190 ) ) ;
#3515=FACE_OUTER_BOUND ( 'NONE', #11111, .T. ) ;
#3518=CARTESIAN_POINT ( 'NONE',  ( -247.5000000000000000, 139.9999999999999716, -126.4213562373078190 ) ) ;
#3520=EDGE_CURVE ( 'NONE', #6950, #4282, #1364, .T. ) ;
#3526=CARTESIAN_POINT ( 'NONE',  ( -372.6100443311099752, 62.67118023337630461, -129.8688800426077705 ) ) ;
#3536=CARTESIAN_POINT ( 'NONE',  ( -374.5804915919682117, 74.30254460433448571, -95.98273762526655162 ) ) ;
#3542=LINE ( 'NONE', #3681, #2143 ) ;
#3547=CARTESIAN_POINT ( 'NONE',  ( -826.3665850287318335, 74.35417337301126395, -106.1988918232330832 ) ) ;
#3549=CARTESIAN_POINT ( 'NONE',  ( -825.1469620822797424, 73.83976809224682825, -142.9404499552402115 ) ) ;
#3552=CARTESIAN_POINT ( 'NONE',  ( -369.8650217330579153, 55.68315087016564036, -123.9032152127662130 ) ) ;
#3554=CARTESIAN_POINT ( 'NONE',  ( -305.0000000000000568, 81.99999999999995737, -89.68077099980384048 ) ) ;
#3556=VECTOR ( 'NONE', #8982, 1000.000000000000000 ) ;
#3557=DIRECTION ( 'NONE',  ( 2.040851148208007875E-17, -1.000000000000000000, -0.000000000000000000 ) ) ;
#3567=CARTESIAN_POINT ( 'NONE',  ( -379.5458574098431654, 101.3607069150075830, -129.8688049444577928 ) ) ;
#3585=VERTEX_POINT ( 'NONE', #11797 ) ;
#3586=EDGE_CURVE ( 'NONE', #864, #9127, #3687, .T. ) ;
#3587=CARTESIAN_POINT ( 'NONE',  ( -372.4126920328553183, 63.14209089232701899, -145.5554648177819388 ) ) ;
#3590=DIRECTION ( 'NONE',  ( -8.163404592832030268E-17, 1.000000000000000000, -0.000000000000000000 ) ) ;
#3592=CIRCLE ( 'NONE', #43, 7.500000000000007105 ) ;
#3593=EDGE_CURVE ( 'NONE', #586, #864, #1530, .T. ) ;
#3604=CARTESIAN_POINT ( 'NONE',  ( -370.1937529848235044, 107.5001225471108626, -132.1631802120997747 ) ) ;
#3610=DIRECTION ( 'NONE',  ( -8.163404592832031500E-17, 1.000000000000000000, 0.000000000000000000 ) ) ;
#3612=CARTESIAN_POINT ( 'NONE',  ( -825.1499223856426397, 73.84923531294184329, -106.4169293550701951 ) ) ;
#3614=CARTESIAN_POINT ( 'NONE',  ( -825.4626643026864485, 73.93730723265402105, -142.9841191000401750 ) ) ;
#3618=DIRECTION ( 'NONE',  ( -0.000000000000000000, -0.000000000000000000, -1.000000000000000000 ) ) ;
#3622=CARTESIAN_POINT ( 'NONE',  ( -247.5000000000000000, 24.00000000000000711, -126.4213562373078190 ) ) ;
#3631=ORIENTED_EDGE ( 'NONE', *, *, #1407, .F. ) ;
#3632=VERTEX_POINT ( 'NONE', #1368 ) ;
#3646=CARTESIAN_POINT ( 'NONE',  ( -372.8197369114613480, 99.38977441760248155, -147.2377432227614520 ) ) ;
#3649=EDGE_CURVE ( 'NONE', #9395, #495, #2950, .T. ) ;
#3659=CARTESIAN_POINT ( 'NONE',  ( -382.1381191270742761, 67.86032419806703331, -138.8291321671420633 ) ) ;
#3664=B_SPLINE_CURVE_WITH_KNOTS ( 'NONE', 3,
 ( #2011, #8744, #1953, #5025, #324, #2191, #11526, #4110, #4793, #11403, #2998, #5833, #8563, #2881, #6703, #84, #2075, #8691, #4846, #8627, #5713, #200, #3055, #5897, #10595, #141, #2135, #6827, #9671, #1209, #5769, #3924, #10655, #7695, #11466, #11593, #3110, #6885, #8859, #1562, #5325, #4165, #3397, #8975, #3225, #2486, #2371, #2421, #7188, #11884, #501, #6201 ),
 .UNSPECIFIED., .F., .F.,
 ( 4, 2, 2, 2, 2, 2, 2, 2, 2, 2, 2, 2, 2, 2, 2, 2, 2, 2, 2, 2, 2, 2, 2, 2, 2, 4 ),
 ( 0.07032306561503316733, 0.07210969465899567943, 0.07389632370295820540, 0.07568295274692071750, 0.07746958179088322960, 0.08104283987880832318, 0.08461609796673341677, 0.08640272701069594274, 0.08818935605465848260, 0.09176261414258357618, 0.09354924318654614379, 0.09444255770852742760, 0.09533587223050871140, 0.09890913031843383274, 0.1006957593623963865, 0.1024823884063589263, 0.1060556464942840477, 0.1078422755382466014, 0.1096289045822091412, 0.1132021626701343042, 0.1149887917140968996, 0.1167754207580594672, 0.1203486788459845747, 0.1221353078899471561, 0.1239219369339097376, 0.1274951950218348451 ),
 .UNSPECIFIED. ) ;
#3666=EDGE_CURVE ( 'NONE', #2997, #90, #8481, .T. ) ;
#3667=ADVANCED_FACE ( 'NONE', ( #1252 ), #2359, .F. ) ;
#3673=CARTESIAN_POINT ( 'NONE',  ( -379.1619848709566440, 102.0000000000000142, -124.6807709998038405 ) ) ;
#3677=CARTESIAN_POINT ( 'NONE',  ( -828.0828412852908968, 81.30646073758796888, -144.6692115456658598 ) ) ;
#3681=CARTESIAN_POINT ( 'NONE',  ( 0.000000000000000000, 81.99999999999995737, -159.6807709998038547 ) ) ;
#3682=LINE ( 'NONE', #9439, #10211 ) ;
#3687=B_SPLINE_CURVE_WITH_KNOTS ( 'NONE', 3,
 ( #4316, #3313, #11856, #9934, #10858, #6233, #9815, #7911 ),
 .UNSPECIFIED., .F., .F.,
 ( 4, 2, 2, 4 ),
 ( 0.06374494753957145321, 0.06538947705843686786, 0.06703400657730228251, 0.07032306561503316733 ),
 .UNSPECIFIED. ) ;
#3688=CARTESIAN_POINT ( 'NONE',  ( -818.9891295040788464, 77.37577012655981434, -105.2199448511378819 ) ) ;
#3690=CARTESIAN_POINT ( 'NONE',  ( -824.6569351206097735, 73.74060470499414066, -142.8957018107298040 ) ) ;
#3692=CARTESIAN_POINT ( 'NONE',  ( -373.6433083154181531, 68.25182830884359930, -150.2667927013042970 ) ) ;
#3693=CARTESIAN_POINT ( 'NONE',  ( -371.5221853768310325, 103.7913954946613728, -107.9473401059475890 ) ) ;
#3699=AXIS2_PLACEMENT_3D ( 'NONE', #6916, #9004, #2284 ) ;
#3704=DIRECTION ( 'NONE',  ( -8.163404592832030268E-17, 1.000000000000000000, -0.000000000000000000 ) ) ;
#3706=CARTESIAN_POINT ( 'NONE',  ( -372.4693655937733183, 101.8286029160101549, -121.6495295015975273 ) ) ;
#3710=ORIENTED_EDGE ( 'NONE', *, *, #9999, .F. ) ;
#3713=CARTESIAN_POINT ( 'NONE',  ( -383.7289910790237855, 91.48765077515149358, -142.2992162448462068 ) ) ;
#3718=ORIENTED_EDGE ( 'NONE', *, *, #5149, .T. ) ;
#3724=FACE_BOUND ( 'NONE', #2034, .T. ) ;
#3727=CARTESIAN_POINT ( 'NONE',  ( -372.4202255147081360, 61.99933121941937486, -123.1818127415012896 ) ) ;
#3732=DIRECTION ( 'NONE',  ( -1.000000000000000000, 0.000000000000000000, 0.000000000000000000 ) ) ;
#3737=CARTESIAN_POINT ( 'NONE',  ( -305.0000000000000568, 81.99999999999995737, -89.68077099980384048 ) ) ;
#3740=ORIENTED_EDGE ( 'NONE', *, *, #6969, .T. ) ;
#3742=EDGE_CURVE ( 'NONE', #2820, #1615, #9430, .T. ) ;
#3748=CARTESIAN_POINT ( 'NONE',  ( -818.8285638327206470, 78.67432280806529832, -264.6807709998040536 ) ) ;
#3750=CARTESIAN_POINT ( 'NONE',  ( -826.9035580923963380, 74.71835857218523813, -106.0523996049646769 ) ) ;
#3752=ORIENTED_EDGE ( 'NONE', *, *, #9016, .T. ) ;
#3753=CARTESIAN_POINT ( 'NONE',  ( -2.775557561562891351E-14, 139.9999999999999716, -159.6807709998038547 ) ) ;
#3759=CARTESIAN_POINT ( 'NONE',  ( -97.50000000000000000, 152.0000000000000000, -126.4213562373088564 ) ) ;
#3766=CYLINDRICAL_SURFACE ( 'NONE', #1968, 7.500000000000007105 ) ;
#3773=CARTESIAN_POINT ( 'NONE',  ( -380.8316613798133403, 98.99442196914210967, -135.2453119940010140 ) ) ;
#3781=EDGE_LOOP ( 'NONE', ( #3990, #2108, #4113, #8285 ) ) ;
#3782=CARTESIAN_POINT ( 'NONE',  ( -375.0054150261470340, 82.02639447815485596, -154.6972847430876925 ) ) ;
#3784=CARTESIAN_POINT ( 'NONE',  ( -374.8879932666449122, 77.11444321722318307, -105.2520959535442557 ) ) ;
#3789=AXIS2_PLACEMENT_3D ( 'NONE', #11053, #11859, #5489 ) ;
#3794=CARTESIAN_POINT ( 'NONE',  ( -7.499999999999994671, -9.213203435596451385, -126.4213562373094959 ) ) ;
#3797=ORIENTED_EDGE ( 'NONE', *, *, #2991, .F. ) ;
#3798=CARTESIAN_POINT ( 'NONE',  ( -819.8521517457879781, 81.72352651608152030, -144.6807563939346437 ) ) ;
#3809=DIRECTION ( 'NONE',  ( 1.000000000000000000, 0.000000000000000000, 0.000000000000000000 ) ) ;
#3811=DIRECTION ( 'NONE',  ( -8.163404592832030268E-17, 1.000000000000000000, -0.000000000000000000 ) ) ;
#3813=CARTESIAN_POINT ( 'NONE',  ( -374.8738968220091010, 87.13760577545254193, -105.3208045665617050 ) ) ;
#3821=CIRCLE ( 'NONE', #4218, 7.500000000000007105 ) ;
#3825=CARTESIAN_POINT ( 'NONE',  ( -365.0000000000000568, 81.99999999999997158, -124.6807709998038405 ) ) ;
#3836=CARTESIAN_POINT ( 'NONE',  ( -372.9336440560613255, 100.1246349412789556, -133.3251676657040150 ) ) ;
#3837=FACE_OUTER_BOUND ( 'NONE', #8759, .T. ) ;
#3845=DIRECTION ( 'NONE',  ( -1.000000000000000000, 0.000000000000000000, 0.000000000000000000 ) ) ;
#3848=CARTESIAN_POINT ( 'NONE',  ( -374.7692102046581795, 75.20231895184195992, -143.5370633296073493 ) ) ;
#3850=CARTESIAN_POINT ( 'NONE',  ( -374.4847994008925980, 73.48375005241382496, -96.28629692668562257 ) ) ;
#3861=ORIENTED_EDGE ( 'NONE', *, *, #391, .T. ) ;
#3863=AXIS2_PLACEMENT_3D ( 'NONE', #2103, #10322, #8538 ) ;
#3865=SHAPE_DEFINITION_REPRESENTATION ( #10383, #6140 ) ;
#3866=CARTESIAN_POINT ( 'NONE',  ( -370.0251988910513887, 107.9185164359716111, -129.9457498366273285 ) ) ;
#3873=DIRECTION ( 'NONE',  ( -1.000000000000000000, 0.000000000000000000, 0.000000000000000000 ) ) ;
#3902=DIRECTION ( 'NONE',  ( 1.000000000000000000, 1.486905836551548832E-16, -0.000000000000000000 ) ) ;
#3904=CARTESIAN_POINT ( 'NONE',  ( -380.8597684633047038, 98.93849339411727328, -135.3307194093575276 ) ) ;
#3907=AXIS2_PLACEMENT_3D ( 'NONE', #4669, #6633, #836 ) ;
#3908=CARTESIAN_POINT ( 'NONE',  ( -375.0012963295443456, 82.01691494583486985, -144.6876712114242594 ) ) ;
#3910=CARTESIAN_POINT ( 'NONE',  ( -373.7553986963736179, 68.76651228785951275, -98.69780169588010210 ) ) ;
#3911=CARTESIAN_POINT ( 'NONE',  ( 35.00000000000000000, 139.9999999999999716, -159.6807709998038547 ) ) ;
#3912=ADVANCED_FACE ( 'NONE', ( #1920 ), #4281, .T. ) ;
#3913=ORIENTED_EDGE ( 'NONE', *, *, #11025, .T. ) ;
#3916=CIRCLE ( 'NONE', #2520, 7.500000000000007105 ) ;
#3924=CARTESIAN_POINT ( 'NONE',  ( -384.1454913942860685, 89.85401471197820911, -106.2499034276999055 ) ) ;
#3925=EDGE_LOOP ( 'NONE', ( #3128, #5014 ) ) ;
#3933=CARTESIAN_POINT ( 'NONE',  ( -59.99999999999998579, -9.213203435596451385, -126.4213562373090696 ) ) ;
#3940=ORIENTED_EDGE ( 'NONE', *, *, #7922, .T. ) ;
#3945=EDGE_CURVE ( 'NONE', #7284, #4621, #7893, .T. ) ;
#3946=LINE ( 'NONE', #5736, #2428 ) ;
#3949=CARTESIAN_POINT ( 'NONE',  ( -818.8602300167369776, 79.32305858693273137, -104.8581405595891169 ) ) ;
#3952=CARTESIAN_POINT ( 'NONE',  ( -380.5110847637466804, 99.61677185140682411, -115.1901175520814462 ) ) ;
#3963=CARTESIAN_POINT ( 'NONE',  ( -381.1761140529453087, 98.29529414878385296, -136.2909970179879906 ) ) ;
#3964=DIRECTION ( 'NONE',  ( 0.000000000000000000, 1.000000000000000000, -0.000000000000000000 ) ) ;
#3967=CARTESIAN_POINT ( 'NONE',  ( -374.7894439079065023, 75.48283603055834590, -143.6333451466693134 ) ) ;
#3968=CARTESIAN_POINT ( 'NONE',  ( -370.4431240880636551, 57.15653990293812825, -114.9924028573050663 ) ) ;
#3969=CARTESIAN_POINT ( 'NONE',  ( -374.9521586694311850, 79.37652290581388570, -94.82683079494582046 ) ) ;
#3971=VERTEX_POINT ( 'NONE', #5798 ) ;
#3983=EDGE_LOOP ( 'NONE', ( #3301, #536 ) ) ;
#3990=ORIENTED_EDGE ( 'NONE', *, *, #1560, .F. ) ;
#3997=CARTESIAN_POINT ( 'NONE',  ( -818.8285638327206470, 78.34163520102097777, -105.0153140909395120 ) ) ;
#3999=CARTESIAN_POINT ( 'NONE',  ( -112.4999999999999716, -9.213203435596451385, -126.4213562373086575 ) ) ;
#4002=ORIENTED_EDGE ( 'NONE', *, *, #12140, .T. ) ;
#4013=CIRCLE ( 'NONE', #5190, 10.00000000000000000 ) ;
#4018=FACE_BOUND ( 'NONE', #6526, .T. ) ;
#4021=LINE ( 'NONE', #301, #1222 ) ;
#4023=CARTESIAN_POINT ( 'NONE',  ( -373.4475746528857485, 67.29758586747009019, -99.77979850356791758 ) ) ;
#4026=ORIENTED_EDGE ( 'NONE', *, *, #9780, .T. ) ;
#4028=CARTESIAN_POINT ( 'NONE',  ( -384.0282500477451322, 90.36076542521846022, -142.8872781659942177 ) ) ;
#4032=AXIS2_PLACEMENT_3D ( 'NONE', #1512, #8015, #516 ) ;
#4035=CARTESIAN_POINT ( 'NONE',  ( -374.9975296411568024, 81.20712878759192677, -144.6676090229494775 ) ) ;
#4039=ORIENTED_EDGE ( 'NONE', *, *, #6516, .T. ) ;
#4044=ADVANCED_FACE ( 'NONE', ( #5985 ), #8032, .F. ) ;
#4048=DIRECTION ( 'NONE',  ( -0.000000000000000000, -0.000000000000000000, -1.000000000000000000 ) ) ;
#4050=ORIENTED_EDGE ( 'NONE', *, *, #3945, .T. ) ;
#4058=EDGE_CURVE ( 'NONE', #7697, #6496, #469, .T. ) ;
#4078=CARTESIAN_POINT ( 'NONE',  ( -822.0624079427799415, 83.35484814232630413, -104.7266156443419050 ) ) ;
#4082=FACE_BOUND ( 'NONE', #9321, .T. ) ;
#4083=ORIENTED_EDGE ( 'NONE', *, *, #1726, .F. ) ;
#4092=LINE ( 'NONE', #7861, #10009 ) ;
#4094=CARTESIAN_POINT ( 'NONE',  ( -382.6758974726718634, 94.76977496699193182, -140.0841047258399215 ) ) ;
#4098=CARTESIAN_POINT ( 'NONE',  ( -380.4977426702656658, 64.35709158751954817, -115.2383737207536427 ) ) ;
#4102=EDGE_LOOP ( 'NONE', ( #9049, #7363 ) ) ;
#4103=ADVANCED_FACE ( 'NONE', ( #6200 ), #323, .F. ) ;
#4104=CIRCLE ( 'NONE', #3302, 69.99999999999998579 ) ;
#4108=ORIENTED_EDGE ( 'NONE', *, *, #8375, .F. ) ;
#4110=CARTESIAN_POINT ( 'NONE',  ( -381.1875678672224694, 65.72850031932472348, -113.0372152455248198 ) ) ;
#4111=ORIENTED_EDGE ( 'NONE', *, *, #4280, .T. ) ;
#4113=ORIENTED_EDGE ( 'NONE', *, *, #8375, .T. ) ;
#4117=CARTESIAN_POINT ( 'NONE',  ( -180.0000000000000000, -9.213203435596478030, -126.4213562373082453 ) ) ;
#4125=VERTEX_POINT ( 'NONE', #4350 ) ;
#4129=DIRECTION ( 'NONE',  ( -1.000000000000000000, 0.000000000000000000, 0.000000000000000000 ) ) ;
#4134=CARTESIAN_POINT ( 'NONE',  ( -819.0908526083424022, 77.06787236046197620, -144.0637517540454553 ) ) ;
#4135=ADVANCED_FACE ( 'NONE', ( #1325 ), #286, .F. ) ;
#4137=DIRECTION ( 'NONE',  ( 0.000000000000000000, 0.000000000000000000, 1.000000000000000000 ) ) ;
#4140=CARTESIAN_POINT ( 'NONE',  ( -372.8331336047301079, 100.5030287243513385, -117.0268099732259515 ) ) ;
#4142=FACE_BOUND ( 'NONE', #10523, .T. ) ;
#4149=ORIENTED_EDGE ( 'NONE', *, *, #11461, .T. ) ;
#4150=DIRECTION ( 'NONE',  ( -8.163404592832031500E-17, 1.000000000000000000, 0.000000000000000000 ) ) ;
#4151=CARTESIAN_POINT ( 'NONE',  ( -383.8834587150378184, 73.10403131824993750, -142.6030770266003742 ) ) ;
#4153=CARTESIAN_POINT ( 'NONE',  ( -375.0000000000000568, 83.44897642188486486, -154.6807709998038831 ) ) ;
#4154=DIRECTION ( 'NONE',  ( 1.000000000000000000, 0.000000000000000000, 0.000000000000000000 ) ) ;
#4165=CARTESIAN_POINT ( 'NONE',  ( -381.0136216353810141, 98.62943157718950715, -113.5542780775817420 ) ) ;
#4169=EDGE_LOOP ( 'NONE', ( #10008, #9035, #7816, #11194 ) ) ;
#4178=EDGE_CURVE ( 'NONE', #10083, #6648, #11019, .T. ) ;
#4184=FACE_OUTER_BOUND ( 'NONE', #8438, .T. ) ;
#4191=CARTESIAN_POINT ( 'NONE',  ( -826.3398728605874339, 83.01019204304883203, -104.7054730589233458 ) ) ;
#4193=CARTESIAN_POINT ( 'NONE',  ( -370.5023963858000684, 106.6873030616109901, -114.4724351692933055 ) ) ;
#4197=CARTESIAN_POINT ( 'NONE',  ( -202.4999999999999716, 12.00000000000001421, -126.4213562373080180 ) ) ;
#4201=CARTESIAN_POINT ( 'NONE',  ( -374.3141123712231320, 72.20286621420174811, -96.83681641041877697 ) ) ;
#4203=DIRECTION ( 'NONE',  ( -8.163404592832030268E-17, 1.000000000000000000, -0.000000000000000000 ) ) ;
#4207=CARTESIAN_POINT ( 'NONE',  ( -383.7473746520292366, 72.58506784310948490, -142.3356691012474755 ) ) ;
#4209=CARTESIAN_POINT ( 'NONE',  ( -372.9446032145285699, 98.87496311769449164, -147.7124752337511779 ) ) ;
#4210=FACE_OUTER_BOUND ( 'NONE', #10593, .T. ) ;
#4211=CARTESIAN_POINT ( 'NONE',  ( -373.9258432311627303, 68.44287225057918533, -109.8786234846105998 ) ) ;
#4214=ORIENTED_EDGE ( 'NONE', *, *, #11025, .F. ) ;
#4216=EDGE_CURVE ( 'NONE', #8861, #5315, #8061, .T. ) ;
#4217=ORIENTED_EDGE ( 'NONE', *, *, #4405, .T. ) ;
#4218=AXIS2_PLACEMENT_3D ( 'NONE', #442, #2321, #9859 ) ;
#4223=CARTESIAN_POINT ( 'NONE',  ( -305.0000000000000568, 11.99999999999998224, -159.6807709998038547 ) ) ;
#4242=CARTESIAN_POINT ( 'NONE',  ( -379.7921418149276747, 63.07164944985365906, -118.2218589048162016 ) ) ;
#4243=CARTESIAN_POINT ( 'NONE',  ( -374.9543748372134360, 85.20913091084348423, -104.9194821374490090 ) ) ;
#4244=VERTEX_POINT ( 'NONE', #10914 ) ;
#4259=CARTESIAN_POINT ( 'NONE',  ( 0.000000000000000000, 12.00000000000001776, -89.68077099980384048 ) ) ;
#4263=CARTESIAN_POINT ( 'NONE',  ( 35.00000000000000000, 139.9999999999999716, -89.68077099980384048 ) ) ;
#4267=CARTESIAN_POINT ( 'NONE',  ( -7.499999999999996447, 12.00000000000001776, -126.4213562373094959 ) ) ;
#4274=CIRCLE ( 'NONE', #932, 7.500000000000007105 ) ;
#4277=CARTESIAN_POINT ( 'NONE',  ( -371.9170445678053625, 102.5500601245914964, -143.3619720575524070 ) ) ;
#4280=EDGE_CURVE ( 'NONE', #6415, #6258, #150, .T. ) ;
#4281=CYLINDRICAL_SURFACE ( 'NONE', #6501, 69.99999999999995737 ) ;
#4282=VERTEX_POINT ( 'NONE', #8081 ) ;
#4284=AXIS2_PLACEMENT_3D ( 'NONE', #2320, #6089, #4357 ) ;
#4293=ORIENTED_EDGE ( 'NONE', *, *, #3087, .F. ) ;
#4294=CARTESIAN_POINT ( 'NONE',  ( -305.0000000000000568, 81.99999999999995737, -159.6807709998038547 ) ) ;
#4295=ORIENTED_EDGE ( 'NONE', *, *, #86, .F. ) ;
#4302=DIRECTION ( 'NONE',  ( -8.163404592832030268E-17, 1.000000000000000000, -0.000000000000000000 ) ) ;
#4314=CARTESIAN_POINT ( 'NONE',  ( -819.3325619471207801, 76.46264315494589425, -143.9014485902359297 ) ) ;
#4316=CARTESIAN_POINT ( 'NONE',  ( -379.1619848709566440, 61.99999999999992184, -124.6807709998039542 ) ) ;
#4319=CYLINDRICAL_SURFACE ( 'NONE', #11022, 7.500000000000007105 ) ;
#4324=CARTESIAN_POINT ( 'NONE',  ( -142.5000000000000000, -9.213203435596451385, -126.4213562373084301 ) ) ;
#4331=CARTESIAN_POINT ( 'NONE',  ( -384.9934929388428486, 81.09111041420437971, -144.6692448832289131 ) ) ;
#4335=CYLINDRICAL_SURFACE ( 'NONE', #9361, 7.499999999999992895 ) ;
#4339=AXIS2_PLACEMENT_3D ( 'NONE', #529, #11853, #9061 ) ;
#4343=ORIENTED_EDGE ( 'NONE', *, *, #7747, .T. ) ;
#4349=EDGE_LOOP ( 'NONE', ( #6557, #11509, #9254, #5865 ) ) ;
#4350=CARTESIAN_POINT ( 'NONE',  ( -142.5000000000000000, 139.9999999999999716, -126.4213562373084301 ) ) ;
#4354=EDGE_CURVE ( 'NONE', #9244, #8918, #11903, .T. ) ;
#4357=DIRECTION ( 'NONE',  ( 0.000000000000000000, 0.000000000000000000, 1.000000000000000000 ) ) ;
#4381=DIRECTION ( 'NONE',  ( -1.000000000000000000, 0.000000000000000000, 0.000000000000000000 ) ) ;
#4385=EDGE_LOOP ( 'NONE', ( #7626, #8238, #8701, #152 ) ) ;
#4404=FACE_BOUND ( 'NONE', #3983, .T. ) ;
#4405=EDGE_CURVE ( 'NONE', #6480, #11420, #10034, .T. ) ;
#4408=CARTESIAN_POINT ( 'NONE',  ( -379.1617638233734624, 61.99874095070342150, -123.3668595883440986 ) ) ;
#4409=DIRECTION ( 'NONE',  ( -8.163404592832030268E-17, 1.000000000000000000, -0.000000000000000000 ) ) ;
#4412=VECTOR ( 'NONE', #111, 1000.000000000000000 ) ;
#4420=DIRECTION ( 'NONE',  ( -8.163404592832031500E-17, 1.000000000000000000, 0.000000000000000000 ) ) ;
#4423=DIRECTION ( 'NONE',  ( -8.163404592832031500E-17, 1.000000000000000000, 0.000000000000000000 ) ) ;
#4436=CARTESIAN_POINT ( 'NONE',  ( -824.4897464405646588, 73.71539350114024103, -142.8842219741773931 ) ) ;
#4438=CARTESIAN_POINT ( 'NONE',  ( -305.0000000000000568, 24.00000000000000711, -89.68077099980384048 ) ) ;
#4444=AXIS2_PLACEMENT_3D ( 'NONE', #4479, #4671, #4611 ) ;
#4445=VECTOR ( 'NONE', #2316, 1000.000000000000000 ) ;
#4446=FACE_OUTER_BOUND ( 'NONE', #5422, .T. ) ;
#4448=CARTESIAN_POINT ( 'NONE',  ( -372.1690766668580750, 62.27098734669634439, -104.8338495486176640 ) ) ;
#4450=ORIENTED_EDGE ( 'NONE', *, *, #6817, .T. ) ;
#4453=DIRECTION ( 'NONE',  ( -0.000000000000000000, -0.000000000000000000, -1.000000000000000000 ) ) ;
#4455=CARTESIAN_POINT ( 'NONE',  ( -370.4401466759219375, 106.8513018378076822, -134.3428354745942102 ) ) ;
#4461=EDGE_CURVE ( 'NONE', #4719, #1969, #3542, .T. ) ;
#4472=CARTESIAN_POINT ( 'NONE',  ( -372.6372986097472904, 62.76969066101212746, -130.2274012109807302 ) ) ;
#4479=CARTESIAN_POINT ( 'NONE',  ( -59.99999999999998579, -9.213203435596451385, -126.4213562373090696 ) ) ;
#4495=DIRECTION ( 'NONE',  ( -0.1216852752136955151, 0.3205457103956290688, 0.9393844481058480911 ) ) ;
#4496=EDGE_CURVE ( 'NONE', #12134, #3288, #92, .T. ) ;
#4504=CARTESIAN_POINT ( 'NONE',  ( -370.6529647798200813, 57.71370879208589599, -136.1226710876236439 ) ) ;
#4514=EDGE_CURVE ( 'NONE', #7319, #1192, #1900, .T. ) ;
#4516=EDGE_CURVE ( 'NONE', #7116, #90, #11536, .T. ) ;
#4519=DIRECTION ( 'NONE',  ( 0.000000000000000000, 1.000000000000000000, 0.000000000000000000 ) ) ;
#4522=CARTESIAN_POINT ( 'NONE',  ( -372.4515014085467897, 101.8909246911471200, -126.9092234254810876 ) ) ;
#4525=CARTESIAN_POINT ( 'NONE',  ( -187.5000000000000000, 139.9999999999999716, -126.4213562373082453 ) ) ;
#4530=CARTESIAN_POINT ( 'NONE',  ( -180.0000000000000000, 24.00000000000001421, -126.4213562373082453 ) ) ;
#4542=CARTESIAN_POINT ( 'NONE',  ( -373.8419305655268090, 67.98320497006626795, -139.0453867504895129 ) ) ;
#4560=LINE ( 'NONE', #3748, #9735 ) ;
#4562=CARTESIAN_POINT ( 'NONE',  ( -821.5852935318491745, 74.19369191907351535, -106.2666214282630790 ) ) ;
#4565=EDGE_CURVE ( 'NONE', #11519, #3632, #9614, .T. ) ;
#4568=CARTESIAN_POINT ( 'NONE',  ( -370.4431240880636551, 57.15653990293812825, -114.9924028573050663 ) ) ;
#4569=CARTESIAN_POINT ( 'NONE',  ( -382.1463966336086173, 96.15313453893932660, -110.4906001672614622 ) ) ;
#4570=EDGE_CURVE ( 'NONE', #3156, #1708, #357, .T. ) ;
#4588=DIRECTION ( 'NONE',  ( 3.061276722312011504E-17, -1.000000000000000000, 0.000000000000000000 ) ) ;
#4589=DIRECTION ( 'NONE',  ( -8.163404592832030268E-17, 1.000000000000000000, -0.000000000000000000 ) ) ;
#4592=CYLINDRICAL_SURFACE ( 'NONE', #9651, 7.500000000000007105 ) ;
#4594=EDGE_CURVE ( 'NONE', #3971, #7586, #9377, .T. ) ;
#4595=ORIENTED_EDGE ( 'NONE', *, *, #4461, .T. ) ;
#4598=EDGE_LOOP ( 'NONE', ( #5883, #3341 ) ) ;
#4606=CARTESIAN_POINT ( 'NONE',  ( -372.9391702816300835, 63.88999388380243261, -133.3467129973068666 ) ) ;
#4607=DIRECTION ( 'NONE',  ( -1.000000000000000000, 0.000000000000000000, 0.000000000000000000 ) ) ;
#4608=FACE_OUTER_BOUND ( 'NONE', #5824, .T. ) ;
#4611=DIRECTION ( 'NONE',  ( -1.000000000000000000, 0.000000000000000000, 0.000000000000000000 ) ) ;
#4613=LINE ( 'NONE', #9482, #11534 ) ;
#4615=DIRECTION ( 'NONE',  ( -1.000000000000000000, 0.000000000000000000, 0.000000000000000000 ) ) ;
#4616=DIRECTION ( 'NONE',  ( -1.000000000000000000, 0.000000000000000000, 0.000000000000000000 ) ) ;
#4617=ORIENTED_EDGE ( 'NONE', *, *, #3077, .F. ) ;
#4618=CARTESIAN_POINT ( 'NONE',  ( -820.0597211274471192, 81.97619047958252736, -144.6820902952096901 ) ) ;
#4620=CARTESIAN_POINT ( 'NONE',  ( -372.4687937583217945, 100.6702782477001819, -103.5591500974845047 ) ) ;
#4621=VERTEX_POINT ( 'NONE', #6651 ) ;
#4629=CARTESIAN_POINT ( 'NONE',  ( -820.0492617104155215, 75.38478674231490118, -105.8049000242699833 ) ) ;
#4633=CIRCLE ( 'NONE', #11922, 7.500000000000007105 ) ;
#4634=EDGE_LOOP ( 'NONE', ( #1677, #9137, #10456, #8973 ) ) ;
#4635=CARTESIAN_POINT ( 'NONE',  ( -371.3925255517432333, 59.81623701251285752, -140.7297140340658927 ) ) ;
#4636=CARTESIAN_POINT ( 'NONE',  ( -374.8878514016580539, 86.86219835938075562, -105.2522987037355477 ) ) ;
#4652=DIRECTION ( 'NONE',  ( -1.000000000000000000, 0.000000000000000000, 0.000000000000000000 ) ) ;
#4655=VERTEX_POINT ( 'NONE', #7945 ) ;
#4657=ORIENTED_EDGE ( 'NONE', *, *, #11211, .T. ) ;
#4660=EDGE_LOOP ( 'NONE', ( #1170, #8764, #5140, #10036 ) ) ;
#4667=CARTESIAN_POINT ( 'NONE',  ( -371.5191645905044879, 60.19565412010540939, -141.4135686812714141 ) ) ;
#4669=CARTESIAN_POINT ( 'NONE',  ( -180.0000000000000000, -9.213203435596478030, -126.4213562373082453 ) ) ;
#4670=( GEOMETRIC_REPRESENTATION_CONTEXT ( 3 ) GLOBAL_UNCERTAINTY_ASSIGNED_CONTEXT ( ( #4916 ) ) GLOBAL_UNIT_ASSIGNED_CONTEXT ( ( #3090, #4938, #11564 ) ) REPRESENTATION_CONTEXT ( 'NONE', 'WORKASPACE' ) );
#4671=DIRECTION ( 'NONE',  ( -8.163404592832030268E-17, 1.000000000000000000, -0.000000000000000000 ) ) ;
#4674=CARTESIAN_POINT ( 'NONE',  ( -305.0000000000000568, 81.99999999999995737, -159.6807709998038547 ) ) ;
#4683=CARTESIAN_POINT ( 'NONE',  ( -822.5351658412957931, 83.51517767605524512, -144.6233963009597687 ) ) ;
#4695=CARTESIAN_POINT ( 'NONE',  ( -828.6675604493455012, 77.37337224769238730, -105.2204629476320719 ) ) ;
#4698=LINE ( 'NONE', #4438, #11123 ) ;
#4710=FACE_OUTER_BOUND ( 'NONE', #2773, .T. ) ;
#4712=VERTEX_POINT ( 'NONE', #5921 ) ;
#4713=CARTESIAN_POINT ( 'NONE',  ( -373.3728075979055347, 98.29427327314448348, -136.3749942106433366 ) ) ;
#4717=AXIS2_PLACEMENT_3D ( 'NONE', #3487, #8335, #11037 ) ;
#4719=VERTEX_POINT ( 'NONE', #10673 ) ;
#4724=CARTESIAN_POINT ( 'NONE',  ( -374.8265083808032045, 76.03942901340127491, -143.8108696807164790 ) ) ;
#4726=CARTESIAN_POINT ( 'NONE',  ( -384.2251555493538717, 74.58855242484294479, -106.1017844575084439 ) ) ;
#4740=CARTESIAN_POINT ( 'NONE',  ( -827.8097080315036465, 81.71711720835109816, -144.6806456489624395 ) ) ;
#4741=CARTESIAN_POINT ( 'NONE',  ( -374.0007123233734774, 93.82451216013637918, -97.86852803052812533 ) ) ;
#4742=ORIENTED_EDGE ( 'NONE', *, *, #8278, .T. ) ;
#4747=CIRCLE ( 'NONE', #1569, 57.99999999999999289 ) ;
#4750=CARTESIAN_POINT ( 'NONE',  ( -374.0392471180470011, 93.65555499067784240, -97.72940670563750132 ) ) ;
#4766=CARTESIAN_POINT ( 'NONE',  ( -371.5064087246056488, 103.8442247300971530, -141.3454260814483519 ) ) ;
#4768=ORIENTED_EDGE ( 'NONE', *, *, #1014, .F. ) ;
#4770=DIRECTION ( 'NONE',  ( 0.000000000000000000, 0.000000000000000000, 1.000000000000000000 ) ) ;
#4771=ORIENTED_EDGE ( 'NONE', *, *, #2605, .F. ) ;
#4772=VECTOR ( 'NONE', #10044, 1000.000000000000000 ) ;
#4773=FACE_OUTER_BOUND ( 'NONE', #7615, .T. ) ;
#4774=ORIENTED_EDGE ( 'NONE', *, *, #9688, .T. ) ;
#4779=VECTOR ( 'NONE', #7101, 1000.000000000000000 ) ;
#4780=CARTESIAN_POINT ( 'NONE',  ( -374.6843874209988599, 75.16053358314040622, -153.7112566340306046 ) ) ;
#4782=CARTESIAN_POINT ( 'NONE',  ( -384.7852612105363619, 78.04101542915444156, -105.0654598586175581 ) ) ;
#4783=DIRECTION ( 'NONE',  ( 1.000000000000000000, 0.000000000000000000, 0.000000000000000000 ) ) ;
#4786=EDGE_CURVE ( 'NONE', #1233, #7767, #5567, .T. ) ;
#4788=DIRECTION ( 'NONE',  ( 2.040851148208007875E-17, -1.000000000000000000, -0.000000000000000000 ) ) ;
#4793=CARTESIAN_POINT ( 'NONE',  ( -381.3501251071949696, 66.06991304680765609, -112.5745157944540864 ) ) ;
#4794=ORIENTED_EDGE ( 'NONE', *, *, #2374, .T. ) ;
#4795=EDGE_CURVE ( 'NONE', #10372, #1988, #1816, .T. ) ;
#4797=CARTESIAN_POINT ( 'NONE',  ( -372.8708942284384307, 99.15106812072066589, -101.9386899173519936 ) ) ;
#4803=FACE_BOUND ( 'NONE', #11708, .T. ) ;
#4807=CARTESIAN_POINT ( 'NONE',  ( -371.7612374550235472, 103.0478591256022014, -106.7472349355403480 ) ) ;
#4808=CIRCLE ( 'NONE', #3214, 7.500000000000007105 ) ;
#4812=CYLINDRICAL_SURFACE ( 'NONE', #3117, 7.500000000000007105 ) ;
#4813=CIRCLE ( 'NONE', #11135, 7.500000000000007105 ) ;
#4817=DIRECTION ( 'NONE',  ( -1.000000000000000000, 0.000000000000000000, 0.000000000000000000 ) ) ;
#4819=DIRECTION ( 'NONE',  ( -1.000000000000000000, 0.000000000000000000, 0.000000000000000000 ) ) ;
#4820=CYLINDRICAL_SURFACE ( 'NONE', #1660, 7.500000000000007994 ) ;
#4822=AXIS2_PLACEMENT_3D ( 'NONE', #979, #11355, #4858 ) ;
#4826=EDGE_LOOP ( 'NONE', ( #849, #11112, #3459, #7940 ) ) ;
#4830=VECTOR ( 'NONE', #10348, 1000.000000000000000 ) ;
#4834=CARTESIAN_POINT ( 'NONE',  ( -374.9996141881664471, 82.89264451733117767, -154.6796575120754653 ) ) ;
#4836=CARTESIAN_POINT ( 'NONE',  ( -382.4095633919862962, 68.53572743257521438, -109.8882287899762389 ) ) ;
#4840=ORIENTED_EDGE ( 'NONE', *, *, #7473, .F. ) ;
#4844=B_SPLINE_CURVE_WITH_KNOTS ( 'NONE', 3,
 ( #9654, #4886, #2178, #181, #3904, #3963, #7732, #2115, #11572, #4094, #1195, #11385, #3035, #243, #4028, #3100, #9712, #5005, #7864, #11638, #5186, #7234, #4331, #10069, #6059, #8893, #8045, #10870, #9826, #4151, #4207, #1366, #7107, #11811, #9892, #2357, #7924, #7982, #3327, #6984, #2406, #10757, #7044, #1427, #5131, #3208, #6245, #11693, #9139, #10999 ),
 .UNSPECIFIED., .F., .F.,
 ( 4, 2, 2, 2, 2, 2, 2, 2, 2, 2, 2, 2, 2, 2, 2, 2, 2, 2, 2, 2, 2, 2, 2, 2, 4 ),
 ( 0.006558949033259317725, 0.01013307393990397348, 0.01192013639322624802, 0.01370719884654851908, 0.01728132375319304040, 0.01906838620651532534, 0.02085544865983761376, 0.02442957356648214895, 0.02621663601980439226, 0.02800369847312663557, 0.03157782337977111525, 0.03336488583309336203, 0.03515194828641559494, 0.03872607319306003298, 0.04051313564638227283, 0.04230019809970450573, 0.04587432300634893684, 0.04766138545967119056, 0.04944844791299343734, 0.05302257281963791702, 0.05480963527296017768, 0.05659669772628243140, 0.05838376017960469205, 0.06017082263292695271, 0.06374494753957145321 ),
 .UNSPECIFIED. ) ;
#4846=CARTESIAN_POINT ( 'NONE',  ( -384.6667163751908447, 76.99832943347863079, -105.2798939677049503 ) ) ;
#4849=EDGE_CURVE ( 'NONE', #3585, #3288, #223, .T. ) ;
#4857=CARTESIAN_POINT ( 'NONE',  ( -59.99999999999998579, 12.00000000000001421, -126.4213562373090696 ) ) ;
#4858=DIRECTION ( 'NONE',  ( -1.000000000000000000, 0.000000000000000000, 0.000000000000000000 ) ) ;
#4860=ORIENTED_EDGE ( 'NONE', *, *, #1726, .T. ) ;
#4863=AXIS2_PLACEMENT_3D ( 'NONE', #11397, #9481, #2068 ) ;
#4865=DIRECTION ( 'NONE',  ( 0.000000000000000000, 0.000000000000000000, 1.000000000000000000 ) ) ;
#4878=CIRCLE ( 'NONE', #3699, 7.500000000000007994 ) ;
#4879=ADVANCED_FACE ( 'NONE', ( #2768 ), #10300, .T. ) ;
#4880=AXIS2_PLACEMENT_3D ( 'NONE', #5955, #1260, #1380 ) ;
#4883=ORIENTED_EDGE ( 'NONE', *, *, #11843, .F. ) ;
#4884=ORIENTED_EDGE ( 'NONE', *, *, #1686, .T. ) ;
#4886=CARTESIAN_POINT ( 'NONE',  ( -380.0073966942719039, 100.5504690541876442, -132.2504864982372226 ) ) ;
#4890=CARTESIAN_POINT ( 'NONE',  ( -384.9269939781261201, 79.69860309749668659, -144.5506590107445390 ) ) ;
#4894=EDGE_CURVE ( 'NONE', #3503, #8380, #2401, .T. ) ;
#4898=ORIENTED_EDGE ( 'NONE', *, *, #8278, .F. ) ;
#4902=CARTESIAN_POINT ( 'NONE',  ( -379.7887390581964837, 100.9343252097582564, -131.1221473163307678 ) ) ;
#4905=ORIENTED_EDGE ( 'NONE', *, *, #3593, .T. ) ;
#4916=UNCERTAINTY_MEASURE_WITH_UNIT (LENGTH_MEASURE( 1.000000000000000082E-05 ), #3090, 'distance_accuracy_value', 'NONE');
#4920=EDGE_LOOP ( 'NONE', ( #9673, #5871 ) ) ;
#4921=CARTESIAN_POINT ( 'NONE',  ( -375.0000000000000568, 81.99999999999994316, -154.6807709998039115 ) ) ;
#4930=ORIENTED_EDGE ( 'NONE', *, *, #5776, .T. ) ;
#4932=EDGE_CURVE ( 'NONE', #11612, #5315, #4021, .T. ) ;
#4938=( NAMED_UNIT ( * ) PLANE_ANGLE_UNIT ( ) SI_UNIT ( $, .RADIAN. ) );
#4946=ORIENTED_EDGE ( 'NONE', *, *, #654, .T. ) ;
#4947=( BOUNDED_SURFACE ( )  B_SPLINE_SURFACE ( 3, 2, ( 
 ( #4455, #11993, #9015 ),
 ( #12055, #7300, #3567 ),
 ( #551, #11866, #3382 ),
 ( #11064, #4522, #2589 ),
 ( #7358, #6361, #10133 ),
 ( #11128, #10940, #5502 ),
 ( #9275, #8360, #51 ),
 ( #878, #3706, #1061 ),
 ( #9580, #6551, #1120 ),
 ( #11200, #7603, #10318 ),
 ( #10267, #1798, #7483 ),
 ( #5622, #294, #10622 ),
 ( #4193, #4140, #9880 ),
 ( #2342, #5860, #7912 ),
 ( #6973, #10742, #9635 ),
 ( #7718, #6048, #3952 ),
 ( #170, #1354, #7784 ),
 ( #11183, #8473, #7529 ),
 ( #3693, #6660, #8346 ),
 ( #10253, #9257, #12234 ),
 ( #4807, #12177, #6718 ),
 ( #36, #5610, #10430 ),
 ( #2832, #1723, #4569 ),
 ( #2896, #1971, #11419 ),
 ( #5483, #5729, #10307 ),
 ( #1047, #7470, #8415 ),
 ( #11296, #801, #102 ),
 ( #2707, #5670, #2775 ),
 ( #9446, #9504, #5550 ),
 ( #4750, #1906, #9324 ),
 ( #8522, #9387, #866 ),
 ( #7648, #3813, #7588 ),
 ( #11358, #4636, #6776 ),
 ( #9802, #5103, #6842 ),
 ( #8643, #11483, #3016 ),
 ( #5273, #4243, #6097 ),
 ( #10845, #3355, #5213 ),
 ( #517, #3411, #1635 ),
 ( #8262, #2497, #1575 ),
 ( #8613, #2872, #8553 ),
 ( #3969, #2121, #7623 ),
 ( #8732, #10583, #132 ),
 ( #8502, #5880, #6632 ),
 ( #72, #2984, #4782 ),
 ( #11391, #8, #1882 ),
 ( #3536, #3784, #2803 ),
 ( #3850, #3041, #9659 ),
 ( #10397, #2930, #4726 ),
 ( #4955, #6746, #6690 ),
 ( #10466, #7559, #5646 ),
 ( #7329, #1940, #6575 ),
 ( #3910, #1200, #7739 ),
 ( #5702, #7684, #2059 ),
 ( #11274, #9476, #2001 ),
 ( #8679, #10340, #5818 ),
 ( #9419, #5758, #9534 ),
 ( #1079, #6812, #4836 ),
 ( #11453, #9596, #187 ),
 ( #11513, #4211, #6876 ),
 ( #9958, #11817, #5246 ),
 ( #7988, #5945, #8791 ),
 ( #11761, #11699, #4098 ),
 ( #3161, #10761, #2295 ),
 ( #6065, #9832, #6151 ),
 ( #7019, #9919, #7139 ),
 ( #1395, #1449, #4242 ) ),
 .UNSPECIFIED., .F., .F., .F. ) 
 B_SPLINE_SURFACE_WITH_KNOTS ( ( 4, 2, 2, 2, 2, 2, 2, 2, 2, 2, 2, 2, 2, 2, 2, 2, 2, 2, 2, 2, 2, 2, 2, 2, 2, 2, 2, 2, 2, 2, 2, 2, 4 ),
 ( 3, 3 ),
 ( 0.000000000000000000, 0.005905868208427481753, 0.008858802312641222629, 0.01181173641685496351, 0.01771760462528244526, 0.01919407167738931830, 0.02067053872949618787, 0.02362347283370992701, 0.02657640693792366615, 0.02805287399003053572, 0.02952934104213740876, 0.03543520925056489052, 0.03838814335477863660, 0.03986461040688550617, 0.04134107745899237574, 0.04724694566741985402, 0.04872341271952672359, 0.05019987977163359316, 0.05315281387584733230, 0.05905868208427481753, 0.06053514913638169403, 0.06201161618848856361, 0.06496455029270230275, 0.06791748439691604189, 0.06939395144902291146, 0.07087041850112978103, 0.07677628670955727319, 0.07825275376166414276, 0.07972922081377101233, 0.08268215491798475147, 0.08858802312641222976, 0.09154095723062596890, 0.09449389133483970804 ),
 ( 0.000000000000000000, 1.000000000000000000 ),
 .UNSPECIFIED. ) 
 GEOMETRIC_REPRESENTATION_ITEM ( )  RATIONAL_B_SPLINE_SURFACE ( (
 ( 1.000000000000000000, 0.8173438319342977154, 1.000000000000000000),
 ( 1.000000000000000000, 0.8219731356928380306, 1.000000000000000000),
 ( 1.000000000000000000, 0.8253030949534714278, 1.000000000000000000),
 ( 1.000000000000000000, 0.8281883099846812923, 1.000000000000000000),
 ( 1.000000000000000000, 0.8287982319878953730, 1.000000000000000000),
 ( 1.000000000000000000, 0.8292799412275436710, 1.000000000000000000),
 ( 1.000000000000000000, 0.8291455057931963468, 1.000000000000000000),
 ( 1.000000000000000000, 0.8276356789430494576, 1.000000000000000000),
 ( 1.000000000000000000, 0.8251732266201541321, 1.000000000000000000),
 ( 1.000000000000000000, 0.8204358190366770609, 1.000000000000000000),
 ( 1.000000000000000000, 0.8194051565372284518, 1.000000000000000000),
 ( 1.000000000000000000, 0.8171807861351056967, 1.000000000000000000),
 ( 1.000000000000000000, 0.8159873918869244847, 1.000000000000000000),
 ( 1.000000000000000000, 0.8122138746351555971, 1.000000000000000000),
 ( 1.000000000000000000, 0.8094285655643660427, 1.000000000000000000),
 ( 1.000000000000000000, 0.8033969199180073240, 1.000000000000000000),
 ( 1.000000000000000000, 0.8001503750370143608, 1.000000000000000000),
 ( 1.000000000000000000, 0.7949907125291132415, 1.000000000000000000),
 ( 1.000000000000000000, 0.7932225112627224739, 1.000000000000000000),
 ( 1.000000000000000000, 0.7895990428243180315, 1.000000000000000000),
 ( 1.000000000000000000, 0.7877388389179781347, 1.000000000000000000),
 ( 1.000000000000000000, 0.7783154489584510616, 1.000000000000000000),
 ( 1.000000000000000000, 0.7703989790022252038, 1.000000000000000000),
 ( 1.000000000000000000, 0.7585783171957931614, 1.000000000000000000),
 ( 1.000000000000000000, 0.7546473462006216826, 1.000000000000000000),
 ( 1.000000000000000000, 0.7488515224148959426, 1.000000000000000000),
 ( 1.000000000000000000, 0.7469324236575801690, 1.000000000000000000),
 ( 1.000000000000000000, 0.7431824754817925038, 1.000000000000000000),
 ( 1.000000000000000000, 0.7413476955835877069, 1.000000000000000000),
 ( 1.000000000000000000, 0.7324082410571595148, 1.000000000000000000),
 ( 1.000000000000000000, 0.7260035404487192867, 1.000000000000000000),
 ( 1.000000000000000000, 0.7194925012805183373, 1.000000000000000000),
 ( 1.000000000000000000, 0.7182652744297027825, 1.000000000000000000),
 ( 1.000000000000000000, 0.7159759613185773253, 1.000000000000000000),
 ( 1.000000000000000000, 0.7149113897941246076, 1.000000000000000000),
 ( 1.000000000000000000, 0.7120188864153280672, 1.000000000000000000),
 ( 1.000000000000000000, 0.7104833412027944384, 1.000000000000000000),
 ( 1.000000000000000000, 0.7071146405918344868, 1.000000000000000000),
 ( 1.000000000000000000, 0.7065236520918728447, 1.000000000000000000),
 ( 1.000000000000000000, 0.7079900934967895409, 1.000000000000000000),
 ( 1.000000000000000000, 0.7083941403342759457, 1.000000000000000000),
 ( 1.000000000000000000, 0.7094079449006509552, 1.000000000000000000),
 ( 1.000000000000000000, 0.7100184007272103415, 1.000000000000000000),
 ( 1.000000000000000000, 0.7121454404538102301, 1.000000000000000000),
 ( 1.000000000000000000, 0.7139577670361945128, 1.000000000000000000),
 ( 1.000000000000000000, 0.7182895641410933507, 1.000000000000000000),
 ( 1.000000000000000000, 0.7208090478352079389, 1.000000000000000000),
 ( 1.000000000000000000, 0.7250557726365194355, 1.000000000000000000),
 ( 1.000000000000000000, 0.7265534932289373637, 1.000000000000000000),
 ( 1.000000000000000000, 0.7296713736093599634, 1.000000000000000000),
 ( 1.000000000000000000, 0.7312892119586734685, 1.000000000000000000),
 ( 1.000000000000000000, 0.7396315842215842595, 1.000000000000000000),
 ( 1.000000000000000000, 0.7471097587475988844, 1.000000000000000000),
 ( 1.000000000000000000, 0.7568743091753726837, 1.000000000000000000),
 ( 1.000000000000000000, 0.7588483787671314040, 1.000000000000000000),
 ( 1.000000000000000000, 0.7628250640091223111, 1.000000000000000000),
 ( 1.000000000000000000, 0.7648239673428672836, 1.000000000000000000),
 ( 1.000000000000000000, 0.7707817864204414837, 1.000000000000000000),
 ( 1.000000000000000000, 0.7747203848179342600, 1.000000000000000000),
 ( 1.000000000000000000, 0.7862853007360839364, 1.000000000000000000),
 ( 1.000000000000000000, 0.7936618350787719711, 1.000000000000000000),
 ( 1.000000000000000000, 0.8036599604343283021, 1.000000000000000000),
 ( 1.000000000000000000, 0.8067667731041444634, 1.000000000000000000),
 ( 1.000000000000000000, 0.8124350975610165060, 1.000000000000000000),
 ( 1.000000000000000000, 0.8150032476531663406, 1.000000000000000000),
 ( 1.000000000000000000, 0.8172789612916436797, 1.000000000000000000) ) ) 
 REPRESENTATION_ITEM ( '' )  SURFACE ( )  );
#4953=CARTESIAN_POINT ( 'NONE',  ( -384.4245930906317881, 88.51370271557355807, -143.6368780726383250 ) ) ;
#4955=CARTESIAN_POINT ( 'NONE',  ( -374.2643749961815729, 71.87048632683526250, -96.99996408687380267 ) ) ;
#4973=DIRECTION ( 'NONE',  ( -8.163404592832030268E-17, 1.000000000000000000, -0.000000000000000000 ) ) ;
#4984=AXIS2_PLACEMENT_3D ( 'NONE', #633, #8001, #11712 ) ;
#4990=CARTESIAN_POINT ( 'NONE',  ( -820.0579670039569464, 81.97422455664136010, -104.6794498541743224 ) ) ;
#5004=EDGE_LOOP ( 'NONE', ( #9906, #7937, #12196, #4108 ) ) ;
#5005=CARTESIAN_POINT ( 'NONE',  ( -384.6502984881886960, 87.01447873645270192, -144.0511302412744499 ) ) ;
#5008=CIRCLE ( 'NONE', #7183, 35.00000000000000000 ) ;
#5010=DIRECTION ( 'NONE',  ( -8.163404592832030268E-17, 1.000000000000000000, -0.000000000000000000 ) ) ;
#5014=ORIENTED_EDGE ( 'NONE', *, *, #4786, .F. ) ;
#5015=EDGE_CURVE ( 'NONE', #2820, #9984, #5990, .T. ) ;
#5024=CARTESIAN_POINT ( 'NONE',  ( -372.5472084145004033, 62.44479106828742232, -120.1925590171575351 ) ) ;
#5025=CARTESIAN_POINT ( 'NONE',  ( -380.2796270122050259, 63.94918908883580144, -116.0487223431423160 ) ) ;
#5046=DIRECTION ( 'NONE',  ( 1.000000000000000000, 0.000000000000000000, 0.000000000000000000 ) ) ;
#5047=CARTESIAN_POINT ( 'NONE',  ( -818.8285638327206470, 78.34153296655567544, -144.3462106687107678 ) ) ;
#5052=FACE_BOUND ( 'NONE', #9824, .T. ) ;
#5064=FACE_BOUND ( 'NONE', #4920, .T. ) ;
#5074=AXIS2_PLACEMENT_3D ( 'NONE', #3450, #4048, #10068 ) ;
#5082=EDGE_CURVE ( 'NONE', #11519, #9164, #6152, .T. ) ;
#5085=CARTESIAN_POINT ( 'NONE',  ( -370.4431240880659288, 57.15653990294408970, -114.9924028572851142 ) ) ;
#5087=EDGE_LOOP ( 'NONE', ( #1151, #8768, #7958, #304 ) ) ;
#5090=EDGE_LOOP ( 'NONE', ( #2013, #9970 ) ) ;
#5096=VECTOR ( 'NONE', #11348, 1000.000000000000000 ) ;
#5100=CARTESIAN_POINT ( 'NONE',  ( -374.4497035394655882, 90.81972200502131898, -96.39717024633597475 ) ) ;
#5103=CARTESIAN_POINT ( 'NONE',  ( -374.9131056416630940, 86.31065638273830132, -105.1272594036523458 ) ) ;
#5119=CARTESIAN_POINT ( 'NONE',  ( -827.6025323198946353, 81.97067649012244317, -104.6794282814518624 ) ) ;
#5121=CIRCLE ( 'NONE', #6296, 20.00000000000008882 ) ;
#5123=CARTESIAN_POINT ( 'NONE',  ( -823.8285638327206470, 78.67432280806529832, -264.6807709998040536 ) ) ;
#5130=EDGE_LOOP ( 'NONE', ( #12006, #6852, #5386, #10778 ) ) ;
#5131=CARTESIAN_POINT ( 'NONE',  ( -379.6799153206045503, 62.87498284247939040, -130.5615721467151786 ) ) ;
#5136=SURFACE_STYLE_FILL_AREA ( #6008 ) ;
#5137=ORIENTED_EDGE ( 'NONE', *, *, #414, .T. ) ;
#5140=ORIENTED_EDGE ( 'NONE', *, *, #165, .F. ) ;
#5149=EDGE_CURVE ( 'NONE', #3632, #3075, #11096, .T. ) ;
#5150=CARTESIAN_POINT ( 'NONE',  ( -172.5000000000000000, 139.9999999999999716, -126.4213562373082453 ) ) ;
#5151=ADVANCED_FACE ( 'NONE', ( #4446 ), #9130, .F. ) ;
#5152=DIRECTION ( 'NONE',  ( -8.163404592832031500E-17, 1.000000000000000000, 0.000000000000000000 ) ) ;
#5155=DIRECTION ( 'NONE',  ( 2.040851148208007875E-17, -1.000000000000000000, -0.000000000000000000 ) ) ;
#5170=ORIENTED_EDGE ( 'NONE', *, *, #2317, .T. ) ;
#5172=CARTESIAN_POINT ( 'NONE',  ( -828.7652305532230912, 79.48420453549654496, -104.8389787515929754 ) ) ;
#5185=ORIENTED_EDGE ( 'NONE', *, *, #7991, .F. ) ;
#5186=CARTESIAN_POINT ( 'NONE',  ( -384.9888944676742426, 83.49078106762718221, -144.6610261000669198 ) ) ;
#5188=DIRECTION ( 'NONE',  ( -8.163404592832030268E-17, 1.000000000000000000, -0.000000000000000000 ) ) ;
#5189=LINE ( 'NONE', #6935, #10639 ) ;
#5190=AXIS2_PLACEMENT_3D ( 'NONE', #8404, #4495, #921 ) ;
#5206=FACE_OUTER_BOUND ( 'NONE', #9640, .T. ) ;
#5213=CARTESIAN_POINT ( 'NONE',  ( -384.8563257790743251, 85.26078067811664596, -104.9374514401265515 ) ) ;
#5226=CARTESIAN_POINT ( 'NONE',  ( -925.0000000000000000, 81.99999999999988631, -124.6807709998038405 ) ) ;
#5229=EDGE_CURVE ( 'NONE', #1988, #10372, #10698, .T. ) ;
#5232=VERTEX_POINT ( 'NONE', #1730 ) ;
#5233=FACE_OUTER_BOUND ( 'NONE', #6829, .T. ) ;
#5235=DIRECTION ( 'NONE',  ( -1.000000000000000000, 0.000000000000000000, 0.000000000000000000 ) ) ;
#5239=ORIENTED_EDGE ( 'NONE', *, *, #11550, .T. ) ;
#5244=CARTESIAN_POINT ( 'NONE',  ( -370.4401466759219375, 106.8513018378076964, -134.3428354745942102 ) ) ;
#5245=DIRECTION ( 'NONE',  ( -0.000000000000000000, 1.000000000000000000, -0.000000000000000000 ) ) ;
#5246=CARTESIAN_POINT ( 'NONE',  ( -381.3731125161232285, 66.09867141544387437, -112.4817134149344184 ) ) ;
#5249=FACE_OUTER_BOUND ( 'NONE', #8605, .T. ) ;
#5258=CARTESIAN_POINT ( 'NONE',  ( -172.5000000000000000, 24.00000000000001421, -126.4213562373082453 ) ) ;
#5260=AXIS2_PLACEMENT_3D ( 'NONE', #66, #9414, #3845 ) ;
#5267=AXIS2_PLACEMENT_3D ( 'NONE', #2221, #9756, #1302 ) ;
#5268=AXIS2_PLACEMENT_3D ( 'NONE', #6576, #5703, #12148 ) ;
#5273=CARTESIAN_POINT ( 'NONE',  ( -374.8169097728642214, 87.13039421098122261, -95.24255214225362920 ) ) ;
#5286=CARTESIAN_POINT ( 'NONE',  ( -819.8405841167650578, 75.64117232352664644, -143.6450765909189329 ) ) ;
#5295=CARTESIAN_POINT ( 'NONE',  ( -370.4431240880636551, 57.15653990293812825, -114.9924028573050663 ) ) ;
#5298=ADVANCED_FACE ( 'NONE', ( #3837 ), #2046, .F. ) ;
#5306=DIRECTION ( 'NONE',  ( -8.163404592832030268E-17, 1.000000000000000000, -0.000000000000000000 ) ) ;
#5315=VERTEX_POINT ( 'NONE', #1990 ) ;
#5322=FACE_BOUND ( 'NONE', #5801, .T. ) ;
#5324=CARTESIAN_POINT ( 'NONE',  ( -379.2145310736904662, 62.08676270979725587, -126.6546628987567402 ) ) ;
#5325=CARTESIAN_POINT ( 'NONE',  ( -381.3375926232646975, 97.95623339593267076, -112.6086769336026663 ) ) ;
#5336=ORIENTED_EDGE ( 'NONE', *, *, #6679, .F. ) ;
#5341=LINE ( 'NONE', #8923, #945 ) ;
#5344=CARTESIAN_POINT ( 'NONE',  ( -379.7887390581964837, 100.9343252097582564, -131.1221473163307678 ) ) ;
#5346=CARTESIAN_POINT ( 'NONE',  ( -823.1660337641022807, 73.70728137675511960, -106.4808805636500324 ) ) ;
#5347=CARTESIAN_POINT ( 'NONE',  ( -828.1715959468207302, 76.17590192436144036, -143.8160639703673098 ) ) ;
#5348=CARTESIAN_POINT ( 'NONE',  ( -825.4402961394276872, 83.41886444745699691, -104.7307635270714314 ) ) ;
#5354=CARTESIAN_POINT ( 'NONE',  ( -210.0000000000000000, 12.00000000000001421, -126.4213562373080180 ) ) ;
#5356=CARTESIAN_POINT ( 'NONE',  ( -127.4999999999999716, -9.213203435596451385, -126.4213562373086575 ) ) ;
#5361=CARTESIAN_POINT ( 'NONE',  ( 0.000000000000000000, 24.00000000000001776, -159.6807709998038547 ) ) ;
#5363=FACE_OUTER_BOUND ( 'NONE', #11938, .T. ) ;
#5364=AXIS2_PLACEMENT_3D ( 'NONE', #9850, #10889, #8058 ) ;
#5365=EDGE_CURVE ( 'NONE', #11420, #6480, #2024, .T. ) ;
#5368=DIRECTION ( 'NONE',  ( -1.000000000000000000, 0.000000000000000000, 0.000000000000000000 ) ) ;
#5380=EDGE_LOOP ( 'NONE', ( #3718, #7921 ) ) ;
#5381=CARTESIAN_POINT ( 'NONE',  ( -370.9998549364893279, 58.67489986252060419, -138.4514685534600460 ) ) ;
#5382=DIRECTION ( 'NONE',  ( 3.061276722312011504E-17, -1.000000000000000000, 0.000000000000000000 ) ) ;
#5386=ORIENTED_EDGE ( 'NONE', *, *, #3262, .T. ) ;
#5400=EDGE_CURVE ( 'NONE', #9244, #586, #7151, .T. ) ;
#5403=DIRECTION ( 'NONE',  ( 0.000000000000000000, -1.000000000000000000, -0.000000000000000000 ) ) ;
#5410=CARTESIAN_POINT ( 'NONE',  ( -828.6674387974358069, 77.37343372931279362, -144.1410586993679033 ) ) ;
#5412=CARTESIAN_POINT ( 'NONE',  ( -370.0965291547436209, 56.26080251570542856, -130.6795707448060853 ) ) ;
#5413=EDGE_LOOP ( 'NONE', ( #4039, #3106, #4883, #1124 ) ) ;
#5420=CARTESIAN_POINT ( 'NONE',  ( -370.7822674372037000, 58.06085559963763387, -112.2852247942253712 ) ) ;
#5422=EDGE_LOOP ( 'NONE', ( #4657, #11251, #1385, #4768 ) ) ;
#5424=B_SPLINE_CURVE_WITH_KNOTS ( 'NONE', 3,
 ( #10800, #5047, #8827, #6109, #9877, #4134, #531, #4314, #7154, #5286, #6231, #9996, #1526, #290, #7466, #11974, #8341, #1649, #6535, #7216, #6342, #6286, #10181, #4436, #3690, #3549, #3614, #8411, #863, #1718, #7405, #2703, #7338, #5347, #11045, #9318, #5410, #597, #11909, #2571, #11179, #1783 ),
 .UNSPECIFIED., .F., .F.,
 ( 4, 2, 2, 2, 2, 2, 2, 2, 2, 2, 2, 2, 2, 2, 2, 2, 2, 2, 2, 2, 4 ),
 ( 0.000000000000000000, 0.0009975002171430115937, 0.001496250325714546230, 0.001995000434286080867, 0.002992500651429167054, 0.003990000868572252807, 0.004987501085715338560, 0.005486251194286759572, 0.005985001302858180584, 0.006982501520001022609, 0.007980001737143863766, 0.008478751845715450444, 0.008977501954287037123, 0.009975002171430533138, 0.01097250238857403262, 0.01197000260571752864, 0.01296750282286102465, 0.01396500304000452240, 0.01496250325714802015, 0.01546125336571982888, 0.01596000347429163760 ),
 .UNSPECIFIED. ) ;
#5426=FACE_BOUND ( 'NONE', #8123, .T. ) ;
#5431=CARTESIAN_POINT ( 'NONE',  ( -2.775557561562891351E-14, 139.9999999999999716, -89.68077099980384048 ) ) ;
#5435=ORIENTED_EDGE ( 'NONE', *, *, #10382, .T. ) ;
#5436=DIRECTION ( 'NONE',  ( 1.000000000000000000, 0.000000000000000000, 0.000000000000000000 ) ) ;
#5444=ORIENTED_EDGE ( 'NONE', *, *, #3077, .T. ) ;
#5445=CARTESIAN_POINT ( 'NONE',  ( -381.0219023890770131, 65.38716504393917717, -135.8359694540845055 ) ) ;
#5447=DIRECTION ( 'NONE',  ( -1.000000000000000000, 0.000000000000000000, 0.000000000000000000 ) ) ;
#5449=AXIS2_PLACEMENT_3D ( 'NONE', #3281, #7057, #9901 ) ;
#5450=FACE_OUTER_BOUND ( 'NONE', #1208, .T. ) ;
#5451=LINE ( 'NONE', #8321, #2088 ) ;
#5452=ADVANCED_FACE ( 'NONE', ( #3263 ), #2352, .F. ) ;
#5454=DIRECTION ( 'NONE',  ( -1.000000000000000000, 0.000000000000000000, 0.000000000000000000 ) ) ;
#5465=EDGE_CURVE ( 'NONE', #3503, #1233, #2227, .T. ) ;
#5476=CARTESIAN_POINT ( 'NONE',  ( -821.2975544693601933, 74.34970510072395200, -106.2007125858225720 ) ) ;
#5477=DIRECTION ( 'NONE',  ( 2.040851148208007875E-17, -1.000000000000000000, -0.000000000000000000 ) ) ;
#5483=CARTESIAN_POINT ( 'NONE',  ( -373.1519908486758368, 97.99425499239711712, -100.8725093751089332 ) ) ;
#5489=DIRECTION ( 'NONE',  ( 1.000000000000000000, 0.000000000000000000, 0.000000000000000000 ) ) ;
#5490=DIRECTION ( 'NONE',  ( -1.000000000000000000, 0.000000000000000000, 0.000000000000000000 ) ) ;
#5491=DIRECTION ( 'NONE',  ( -8.163404592832031500E-17, 1.000000000000000000, 0.000000000000000000 ) ) ;
#5495=ORIENTED_EDGE ( 'NONE', *, *, #11065, .T. ) ;
#5500=LINE ( 'NONE', #2651, #8184 ) ;
#5502=CARTESIAN_POINT ( 'NONE',  ( -379.1553463010024529, 102.0109503771648605, -124.6625911296856088 ) ) ;
#5508=CARTESIAN_POINT ( 'NONE',  ( -374.1876840878753683, 94.02523439044611564, -140.7929094221022979 ) ) ;
#5517=CARTESIAN_POINT ( 'NONE',  ( -379.1358231506008565, 61.95672027140099658, -124.6842552236176687 ) ) ;
#5522=ORIENTED_EDGE ( 'NONE', *, *, #1344, .T. ) ;
#5527=LINE ( 'NONE', #6272, #12071 ) ;
#5531=CARTESIAN_POINT ( 'NONE',  ( -827.1410867119011527, 82.43389265416584522, -144.6774099844741670 ) ) ;
#5534=CARTESIAN_POINT ( 'NONE',  ( -370.2891325637493196, 107.2458676303090925, -116.4427368508418823 ) ) ;
#5542=DIRECTION ( 'NONE',  ( 0.000000000000000000, 0.000000000000000000, 1.000000000000000000 ) ) ;
#5548=CARTESIAN_POINT ( 'NONE',  ( -372.2568423259174892, 62.53082544746772697, -144.9467117470782114 ) ) ;
#5550=CARTESIAN_POINT ( 'NONE',  ( -383.4981472370314464, 92.28971772028073417, -107.5277044879749155 ) ) ;
#5558=ORIENTED_EDGE ( 'NONE', *, *, #8202, .T. ) ;
#5559=CARTESIAN_POINT ( 'NONE',  ( -52.49999999999997868, 24.00000000000001421, -126.4213562373090696 ) ) ;
#5567=CIRCLE ( 'NONE', #3004, 7.500000000000007105 ) ;
#5568=CARTESIAN_POINT ( 'NONE',  ( -374.4727959898146423, 91.87416495705461728, -142.1456732492470394 ) ) ;
#5581=CARTESIAN_POINT ( 'NONE',  ( -370.4278987528730909, 57.11177549475814175, -134.4195693297641014 ) ) ;
#5584=AXIS2_PLACEMENT_3D ( 'NONE', #2941, #10411, #7818 ) ;
#5591=DIRECTION ( 'NONE',  ( -1.000000000000000000, -8.163404592832031500E-17, 0.000000000000000000 ) ) ;
#5595=CARTESIAN_POINT ( 'NONE',  ( -818.8602280653254866, 79.32430977885819345, -144.5036099591915502 ) ) ;
#5597=CARTESIAN_POINT ( 'NONE',  ( -370.0989827543548927, 107.7329936528643657, -118.6480030875499097 ) ) ;
#5610=CARTESIAN_POINT ( 'NONE',  ( -373.8485616844952801, 96.00934940626343916, -110.2553559621317589 ) ) ;
#5622=CARTESIAN_POINT ( 'NONE',  ( -370.4476841044511275, 106.8318587325821341, -114.9410180965496977 ) ) ;
#5624=CARTESIAN_POINT ( 'NONE',  ( -262.5000000000000000, -9.213203435596478030, -126.4213562373076059 ) ) ;
#5627=DIRECTION ( 'NONE',  ( 0.000000000000000000, 0.000000000000000000, 1.000000000000000000 ) ) ;
#5628=ORIENTED_EDGE ( 'NONE', *, *, #2231, .T. ) ;
#5631=CARTESIAN_POINT ( 'NONE',  ( -374.0189381182528905, 95.05895014862441883, -139.9740603887058228 ) ) ;
#5640=PLANE ( 'NONE',  #2130 ) ;
#5644=CARTESIAN_POINT ( 'NONE',  ( -374.2711669801677772, 71.91685023077710071, -152.3836689249183678 ) ) ;
#5645=CARTESIAN_POINT ( 'NONE',  ( -240.0000000000000000, -9.213203435596478030, -126.4213562373078190 ) ) ;
#5646=CARTESIAN_POINT ( 'NONE',  ( -384.0215091375642373, 73.67838221987805980, -106.4912323260315787 ) ) ;
#5655=CIRCLE ( 'NONE', #5449, 7.500000000000020428 ) ;
#5657=ORIENTED_EDGE ( 'NONE', *, *, #4058, .T. ) ;
#5658=CARTESIAN_POINT ( 'NONE',  ( -828.3216978517729103, 80.87401637003858923, -144.6495766896180442 ) ) ;
#5660=CARTESIAN_POINT ( 'NONE',  ( -373.7386929379060234, 95.23712357076890100, -98.76709413358776146 ) ) ;
#5669=FACE_OUTER_BOUND ( 'NONE', #3111, .T. ) ;
#5670=CARTESIAN_POINT ( 'NONE',  ( -374.5417925368921601, 91.27339439224303419, -106.8924592036498638 ) ) ;
#5684=EDGE_CURVE ( 'NONE', #495, #9395, #3391, .T. ) ;
#5685=CARTESIAN_POINT ( 'NONE',  ( -383.5692087195515683, 92.05770259072330930, -141.9802856064553396 ) ) ;
#5689=DIRECTION ( 'NONE',  ( 0.000000000000000000, 1.000000000000000000, -0.000000000000000000 ) ) ;
#5690=VECTOR ( 'NONE', #2085, 1000.000000000000000 ) ;
#5700=CARTESIAN_POINT ( 'NONE',  ( -374.6542199234099826, 73.81176977798163819, -142.9951582143055475 ) ) ;
#5702=CARTESIAN_POINT ( 'NONE',  ( -373.4583060517632020, 67.32383868152314221, -99.73118028973054550 ) ) ;
#5703=DIRECTION ( 'NONE',  ( -8.163404592832030268E-17, 1.000000000000000000, -0.000000000000000000 ) ) ;
#5706=DIRECTION ( 'NONE',  ( 0.000000000000000000, 0.000000000000000000, 1.000000000000000000 ) ) ;
#5709=CIRCLE ( 'NONE', #1373, 7.500000000000007105 ) ;
#5711=DIRECTION ( 'NONE',  ( 2.040851148208007875E-17, -1.000000000000000000, -0.000000000000000000 ) ) ;
#5713=CARTESIAN_POINT ( 'NONE',  ( -384.9053341376281310, 79.33775245455765912, -104.8495957246331898 ) ) ;
#5715=CARTESIAN_POINT ( 'NONE',  ( -828.5766943389837706, 80.27470094935036116, -144.6085013259155687 ) ) ;
#5721=DIRECTION ( 'NONE',  ( -1.000000000000000000, 0.000000000000000000, 0.000000000000000000 ) ) ;
#5722=CARTESIAN_POINT ( 'NONE',  ( -371.2050310453320776, 59.26189320158484009, -109.6722046579261161 ) ) ;
#5725=FACE_BOUND ( 'NONE', #8661, .T. ) ;
#5727=ORIENTED_EDGE ( 'NONE', *, *, #2231, .F. ) ;
#5728=CARTESIAN_POINT ( 'NONE',  ( 0.000000000000000000, 24.00000000000001776, -89.68077099980384048 ) ) ;
#5729=CARTESIAN_POINT ( 'NONE',  ( -374.3412718121057310, 92.91798692285432537, -107.8362180080072363 ) ) ;
#5736=CARTESIAN_POINT ( 'NONE',  ( -232.4999999999999716, -9.213203435596478030, -126.4213562373078190 ) ) ;
#5738=CARTESIAN_POINT ( 'NONE',  ( -150.0000000000000000, 139.9999999999999716, -126.4213562373084301 ) ) ;
#5746=CARTESIAN_POINT ( 'NONE',  ( -373.7480576296653112, 95.20073465036217897, -150.6300429098349980 ) ) ;
#5753=FACE_BOUND ( 'NONE', #9239, .T. ) ;
#5755=CARTESIAN_POINT ( 'NONE',  ( -374.8433861704153855, 76.31617881061603725, -143.8923350075967278 ) ) ;
#5757=CARTESIAN_POINT ( 'NONE',  ( 9.796085511398436814E-16, 152.0000000000000000, -126.4213562373094959 ) ) ;
#5758=CARTESIAN_POINT ( 'NONE',  ( -374.1800622106637775, 69.98049622810512460, -108.6123104269852035 ) ) ;
#5767=ADVANCED_FACE ( 'NONE', ( #1152 ), #8802, .F. ) ;
#5769=CARTESIAN_POINT ( 'NONE',  ( -384.4631009414320033, 88.19375710871752005, -105.6549207029757582 ) ) ;
#5772=ORIENTED_EDGE ( 'NONE', *, *, #5015, .F. ) ;
#5774=VERTEX_POINT ( 'NONE', #7635 ) ;
#5776=EDGE_CURVE ( 'NONE', #9127, #8918, #3664, .T. ) ;
#5777=DIRECTION ( 'NONE',  ( -1.000000000000000000, 0.000000000000000000, 0.000000000000000000 ) ) ;
#5788=ADVANCED_FACE ( 'NONE', ( #3171 ), #9094, .F. ) ;
#5790=AXIS2_PLACEMENT_3D ( 'NONE', #5757, #9533, #1078 ) ;
#5797=ADVANCED_FACE ( 'NONE', ( #1502 ), #7125, .F. ) ;
#5798=CARTESIAN_POINT ( 'NONE',  ( -52.49999999999999289, 139.9999999999999716, -126.4213562373090696 ) ) ;
#5799=DIRECTION ( 'NONE',  ( -1.000000000000000000, 0.000000000000000000, 0.000000000000000000 ) ) ;
#5801=EDGE_LOOP ( 'NONE', ( #785, #5727 ) ) ;
#5804=AXIS2_PLACEMENT_3D ( 'NONE', #5907, #2086, #330 ) ;
#5807=CARTESIAN_POINT ( 'NONE',  ( -305.0000000000000568, 81.99999999999995737, -159.6807709998038547 ) ) ;
#5813=FACE_BOUND ( 'NONE', #10553, .T. ) ;
#5815=ORIENTED_EDGE ( 'NONE', *, *, #1407, .T. ) ;
#5816=CARTESIAN_POINT ( 'NONE',  ( -374.9580429156226842, 78.77578507266967733, -144.4605282461973275 ) ) ;
#5818=CARTESIAN_POINT ( 'NONE',  ( -382.6913354005332621, 69.27723932749148616, -109.2458039676438091 ) ) ;
#5820=ORIENTED_EDGE ( 'NONE', *, *, #10228, .F. ) ;
#5824=EDGE_LOOP ( 'NONE', ( #8490, #8112, #8416, #12092 ) ) ;
#5832=VECTOR ( 'NONE', #6001, 1000.000000000000000 ) ;
#5833=CARTESIAN_POINT ( 'NONE',  ( -382.8521778068924277, 69.69159708733664615, -108.8740338450474923 ) ) ;
#5834=VERTEX_POINT ( 'NONE', #4223 ) ;
#5841=DIRECTION ( 'NONE',  ( -8.163404592832030268E-17, 1.000000000000000000, -0.000000000000000000 ) ) ;
#5842=EDGE_CURVE ( 'NONE', #4282, #6950, #11107, .T. ) ;
#5853=ADVANCED_FACE ( 'NONE', ( #9969 ), #6138, .F. ) ;
#5856=VECTOR ( 'NONE', #2888, 1000.000000000000000 ) ;
#5860=CARTESIAN_POINT ( 'NONE',  ( -372.9463709484128913, 100.0680782940595748, -116.0142139199710130 ) ) ;
#5865=ORIENTED_EDGE ( 'NONE', *, *, #6817, .F. ) ;
#5866=CYLINDRICAL_SURFACE ( 'NONE', #7168, 69.99999999999995737 ) ;
#5871=ORIENTED_EDGE ( 'NONE', *, *, #4795, .F. ) ;
#5873=ORIENTED_EDGE ( 'NONE', *, *, #10530, .F. ) ;
#5874=PLANE ( 'NONE',  #9952 ) ;
#5878=CARTESIAN_POINT ( 'NONE',  ( -383.7345387547151745, 72.53406450605939426, -142.3107974752694531 ) ) ;
#5880=CARTESIAN_POINT ( 'NONE',  ( -374.9733877151688262, 79.55905688470338077, -104.8208928575475767 ) ) ;
#5883=ORIENTED_EDGE ( 'NONE', *, *, #4216, .F. ) ;
#5884=AXIS2_PLACEMENT_3D ( 'NONE', #3027, #11728, #10732 ) ;
#5894=APPLICATION_CONTEXT ( 'automotive_design' ) ;
#5897=CARTESIAN_POINT ( 'NONE',  ( -384.9908864334298642, 81.14062117122209372, -104.6969719710837268 ) ) ;
#5907=CARTESIAN_POINT ( 'NONE',  ( -89.99999999999998579, -9.213203435596451385, -126.4213562373088564 ) ) ;
#5910=FACE_BOUND ( 'NONE', #4102, .T. ) ;
#5913=ORIENTED_EDGE ( 'NONE', *, *, #4058, .F. ) ;
#5914=CARTESIAN_POINT ( 'NONE',  ( -374.9931058222078377, 80.86295360366069929, -154.6597799724412710 ) ) ;
#5916=AXIS2_PLACEMENT_3D ( 'NONE', #4857, #7581, #3873 ) ;
#5920=CARTESIAN_POINT ( 'NONE',  ( -22.49999999999997868, -9.213203435596451385, -126.4213562373092685 ) ) ;
#5921=CARTESIAN_POINT ( 'NONE',  ( -112.4999999999999716, 24.00000000000001421, -126.4213562373086575 ) ) ;
#5925=CARTESIAN_POINT ( 'NONE',  ( -818.8285638327205334, 79.00074005404771071, -104.9041682110412239 ) ) ;
#5929=DIRECTION ( 'NONE',  ( 3.061276722312011504E-17, -1.000000000000000000, 0.000000000000000000 ) ) ;
#5940=CARTESIAN_POINT ( 'NONE',  ( 35.00000000000000000, 152.0000000000000000, -89.68077099980384048 ) ) ;
#5945=CARTESIAN_POINT ( 'NONE',  ( -373.4675643629642536, 66.11521760855615071, -112.3653755622224111 ) ) ;
#5947=( NAMED_UNIT ( * ) SI_UNIT ( $, .STERADIAN. ) SOLID_ANGLE_UNIT ( ) );
#5955=CARTESIAN_POINT ( 'NONE',  ( 1.414009460465297036E-14, -9.213203435596451385, -126.4213562373094959 ) ) ;
#5960=DIRECTION ( 'NONE',  ( 0.000000000000000000, 1.000000000000000000, -0.000000000000000000 ) ) ;
#5961=ORIENTED_EDGE ( 'NONE', *, *, #121, .T. ) ;
#5964=AXIS2_PLACEMENT_3D ( 'NONE', #8222, #9197, #5235 ) ;
#5966=CARTESIAN_POINT ( 'NONE',  ( -89.99999999999998579, -9.213203435596451385, -126.4213562373088564 ) ) ;
#5969=DIRECTION ( 'NONE',  ( 1.486905836551548832E-16, -1.000000000000000000, 0.000000000000000000 ) ) ;
#5981=CARTESIAN_POINT ( 'NONE',  ( -97.50000000000000000, 139.9999999999999716, -126.4213562373088564 ) ) ;
#5984=DIRECTION ( 'NONE',  ( 0.000000000000000000, 1.000000000000000000, -0.000000000000000000 ) ) ;
#5985=FACE_OUTER_BOUND ( 'NONE', #9525, .T. ) ;
#5986=PLANE ( 'NONE',  #10368 ) ;
#5989=DIRECTION ( 'NONE',  ( -0.000000000000000000, -0.000000000000000000, -1.000000000000000000 ) ) ;
#5990=LINE ( 'NONE', #363, #4779 ) ;
#5992=CIRCLE ( 'NONE', #9943, 69.99999999999998579 ) ;
#5996=ORIENTED_EDGE ( 'NONE', *, *, #8202, .F. ) ;
#5997=ORIENTED_EDGE ( 'NONE', *, *, #7440, .T. ) ;
#5999=FACE_BOUND ( 'NONE', #4598, .T. ) ;
#6001=DIRECTION ( 'NONE',  ( -8.163404592832030268E-17, 1.000000000000000000, -0.000000000000000000 ) ) ;
#6008=FILL_AREA_STYLE ('',( #7929 ) ) ;
#6012=CIRCLE ( 'NONE', #6795, 7.500000000000007105 ) ;
#6014=EDGE_CURVE ( 'NONE', #1192, #4655, #3592, .T. ) ;
#6024=ADVANCED_FACE ( 'NONE', ( #9161 ), #11273, .F. ) ;
#6025=ADVANCED_FACE ( 'NONE', ( #8250 ), #697, .F. ) ;
#6036=CARTESIAN_POINT ( 'NONE',  ( 1.240837498110468453E-14, 12.00000000000001776, -126.4213562373094959 ) ) ;
#6048=CARTESIAN_POINT ( 'NONE',  ( -373.1999217634634078, 99.04079563999313507, -114.1166220202556616 ) ) ;
#6051=DIRECTION ( 'NONE',  ( 1.000000000000000000, 0.000000000000000000, 0.000000000000000000 ) ) ;
#6052=ORIENTED_EDGE ( 'NONE', *, *, #7693, .F. ) ;
#6053=PLANE ( 'NONE',  #5267 ) ;
#6059=CARTESIAN_POINT ( 'NONE',  ( -384.9016521429225577, 79.29180104530665574, -144.5054763653512850 ) ) ;
#6065=CARTESIAN_POINT ( 'NONE',  ( -370.6647493025599260, 57.74548308484566661, -113.1662857576497174 ) ) ;
#6069=FACE_OUTER_BOUND ( 'NONE', #637, .T. ) ;
#6070=ORIENTED_EDGE ( 'NONE', *, *, #1014, .T. ) ;
#6081=CARTESIAN_POINT ( 'NONE',  ( -30.00000000000000000, 139.9999999999999716, -126.4213562373092685 ) ) ;
#6089=DIRECTION ( 'NONE',  ( 0.000000000000000000, 1.000000000000000000, -0.000000000000000000 ) ) ;
#6097=CARTESIAN_POINT ( 'NONE',  ( -384.7907540261165309, 85.90887177978304123, -105.0552917614837867 ) ) ;
#6108=DIRECTION ( 'NONE',  ( -1.000000000000000000, 0.000000000000000000, 0.000000000000000000 ) ) ;
#6109=CARTESIAN_POINT ( 'NONE',  ( -818.9567516184583837, 77.53771799247171259, -144.1773011583834716 ) ) ;
#6114=AXIS2_PLACEMENT_3D ( 'NONE', #402, #7028, #6108 ) ;
#6121=CARTESIAN_POINT ( 'NONE',  ( -374.9888490819218987, 80.55335064010526480, -94.71470242688155849 ) ) ;
#6129=CARTESIAN_POINT ( 'NONE',  ( -818.8285638327206470, 78.67432280806531253, -104.9592124606049879 ) ) ;
#6138=CYLINDRICAL_SURFACE ( 'NONE', #6959, 7.500000000000007105 ) ;
#6140=SHAPE_REPRESENTATION ( 'Long Manual Ratchet Lever Handle', ( #11957 ), #4670 ) ;
#6148=DIRECTION ( 'NONE',  ( -0.000000000000000000, -1.000000000000000000, 0.000000000000000000 ) ) ;
#6149=LINE ( 'NONE', #9916, #3556 ) ;
#6151=CARTESIAN_POINT ( 'NONE',  ( -380.0454277744337332, 63.52036806465107333, -117.0044475050485744 ) ) ;
#6152=CIRCLE ( 'NONE', #7735, 7.500000000000007105 ) ;
#6153=VERTEX_POINT ( 'NONE', #11390 ) ;
#6165=CARTESIAN_POINT ( 'NONE',  ( -60.00000000000000000, 139.9999999999999716, -126.4213562373090696 ) ) ;
#6170=CARTESIAN_POINT ( 'NONE',  ( -827.1368241426257555, 82.43785830827043526, -104.6842000310832503 ) ) ;
#6175=AXIS2_PLACEMENT_3D ( 'NONE', #10152, #1689, #5447 ) ;
#6186=DIRECTION ( 'NONE',  ( -1.000000000000000000, 0.000000000000000000, 0.000000000000000000 ) ) ;
#6187=LINE ( 'NONE', #9955, #7777 ) ;
#6191=VERTEX_POINT ( 'NONE', #3968 ) ;
#6192=DIRECTION ( 'NONE',  ( 1.000000000000000000, 0.000000000000000000, 0.000000000000000000 ) ) ;
#6200=FACE_OUTER_BOUND ( 'NONE', #7017, .T. ) ;
#6201=CARTESIAN_POINT ( 'NONE',  ( -379.1619848709566440, 102.0000000000000142, -124.6807709998038405 ) ) ;
#6203=CARTESIAN_POINT ( 'NONE',  ( -127.5000000000000000, 152.0000000000000000, -126.4213562373086575 ) ) ;
#6207=CIRCLE ( 'NONE', #6408, 7.500000000000007105 ) ;
#6210=CARTESIAN_POINT ( 'NONE',  ( 1.142876642996484321E-14, 24.00000000000001421, -126.4213562373094959 ) ) ;
#6222=CARTESIAN_POINT ( 'NONE',  ( -180.0000000000000000, 151.9999999999999716, -126.4213562373082453 ) ) ;
#6226=EDGE_CURVE ( 'NONE', #5315, #8861, #10148, .T. ) ;
#6229=EDGE_CURVE ( 'NONE', #4655, #1192, #451, .T. ) ;
#6231=CARTESIAN_POINT ( 'NONE',  ( -820.0477536417059810, 75.38653579115350567, -143.5572547269224515 ) ) ;
#6233=CARTESIAN_POINT ( 'NONE',  ( -379.4351561318256358, 62.45525130393783542, -120.2966889111102660 ) ) ;
#6234=ORIENTED_EDGE ( 'NONE', *, *, #10821, .F. ) ;
#6241=DIRECTION ( 'NONE',  ( 0.000000000000000000, 1.000000000000000000, 0.000000000000000000 ) ) ;
#6242=ORIENTED_EDGE ( 'NONE', *, *, #11755, .F. ) ;
#6245=CARTESIAN_POINT ( 'NONE',  ( -379.4184094136624594, 62.42756673384518962, -128.8379558659856059 ) ) ;
#6258=VERTEX_POINT ( 'NONE', #3040 ) ;
#6262=CARTESIAN_POINT ( 'NONE',  ( -380.4284056416585713, 64.22849513334448091, -133.8612360355819817 ) ) ;
#6272=CARTESIAN_POINT ( 'NONE',  ( 35.00000000000000000, 152.0000000000000000, -159.6807709998038547 ) ) ;
#6277=CARTESIAN_POINT ( 'NONE',  ( -305.0000000000000568, 12.00000000000001066, -159.6807709998038547 ) ) ;
#6285=CARTESIAN_POINT ( 'NONE',  ( -824.5038201930738069, 73.70910806073447930, -106.4800466717824037 ) ) ;
#6286=CARTESIAN_POINT ( 'NONE',  ( -823.9892610140070701, 73.67413949648553739, -142.8653811665924991 ) ) ;
#6296=AXIS2_PLACEMENT_3D ( 'NONE', #5226, #3251, #8997 ) ;
#6301=DIRECTION ( 'NONE',  ( -8.163404592832030268E-17, 1.000000000000000000, -0.000000000000000000 ) ) ;
#6303=ADVANCED_FACE ( 'NONE', ( #4210 ), #4335, .F. ) ;
#6322=CARTESIAN_POINT ( 'NONE',  ( -372.4518007995145013, 62.11038424318570605, -126.9228541902815692 ) ) ;
#6330=CIRCLE ( 'NONE', #828, 7.500000000000007105 ) ;
#6337=DIRECTION ( 'NONE',  ( 1.000000000000000000, 1.486905836551548832E-16, -0.000000000000000000 ) ) ;
#6340=CARTESIAN_POINT ( 'NONE',  ( -827.6116171724344213, 75.38904402456984144, -105.8033998852342421 ) ) ;
#6342=CARTESIAN_POINT ( 'NONE',  ( -823.4903519156962375, 73.67469885889892112, -142.8656372648659953 ) ) ;
#6344=ORIENTED_EDGE ( 'NONE', *, *, #2675, .F. ) ;
#6345=CARTESIAN_POINT ( 'NONE',  ( -370.0925635847275998, 56.25177319444339474, -118.8156198848447787 ) ) ;
#6348=CARTESIAN_POINT ( 'NONE',  ( -187.5000000000000000, 12.00000000000001421, -126.4213562373082453 ) ) ;
#6352=CARTESIAN_POINT ( 'NONE',  ( -247.5000000000000000, -9.213203435596478030, -126.4213562373078190 ) ) ;
#6356=ORIENTED_EDGE ( 'NONE', *, *, #9016, .F. ) ;
#6361=CARTESIAN_POINT ( 'NONE',  ( -372.4316250286643140, 101.9596924382562122, -126.1642065034420028 ) ) ;
#6366=VERTEX_POINT ( 'NONE', #6934 ) ;
#6370=VERTEX_POINT ( 'NONE', #9831 ) ;
#6377=EDGE_CURVE ( 'NONE', #3075, #3632, #4633, .T. ) ;
#6382=CARTESIAN_POINT ( 'NONE',  ( -373.3345058608713316, 65.54065180381869027, -136.1221809958202300 ) ) ;
#6385=ORIENTED_EDGE ( 'NONE', *, *, #5082, .F. ) ;
#6388=EDGE_CURVE ( 'NONE', #5232, #10372, #7869, .T. ) ;
#6393=DIRECTION ( 'NONE',  ( -1.000000000000000000, 0.000000000000000000, 0.000000000000000000 ) ) ;
#6398=CARTESIAN_POINT ( 'NONE',  ( -819.3316697785950282, 80.88429704961208699, -144.6519063719966027 ) ) ;
#6399=AXIS2_PLACEMENT_3D ( 'NONE', #7046, #3160, #2237 ) ;
#6405=DIRECTION ( 'NONE',  ( -8.163404592832030268E-17, 1.000000000000000000, -0.000000000000000000 ) ) ;
#6406=EDGE_CURVE ( 'NONE', #9394, #546, #8175, .T. ) ;
#6408=AXIS2_PLACEMENT_3D ( 'NONE', #7825, #210, #11476 ) ;
#6409=CARTESIAN_POINT ( 'NONE',  ( -823.8285638327206470, 78.67432280806529832, -264.6807709998040536 ) ) ;
#6415=VERTEX_POINT ( 'NONE', #2473 ) ;
#6420=DIRECTION ( 'NONE',  ( -8.163404592832031500E-17, 1.000000000000000000, 0.000000000000000000 ) ) ;
#6422=CARTESIAN_POINT ( 'NONE',  ( -371.4336752585604700, 59.93884798725025576, -108.4060072831181714 ) ) ;
#6425=ORIENTED_EDGE ( 'NONE', *, *, #1761, .T. ) ;
#6430=CARTESIAN_POINT ( 'NONE',  ( -29.99999999999998579, -9.213203435596451385, -126.4213562373092685 ) ) ;
#6434=CARTESIAN_POINT ( 'NONE',  ( -270.0000000000000000, -9.213203435596478030, -126.4213562373076059 ) ) ;
#6437=CARTESIAN_POINT ( 'NONE',  ( -373.5257043960141914, 96.29568266366972296, -149.8465111201311686 ) ) ;
#6448=CARTESIAN_POINT ( 'NONE',  ( -372.4958542361324589, 63.44167550995515370, -145.9033127508436962 ) ) ;
#6451=EDGE_CURVE ( 'NONE', #6496, #2042, #2410, .T. ) ;
#6452=DIRECTION ( 'NONE',  ( -0.000000000000000000, -0.000000000000000000, -1.000000000000000000 ) ) ;
#6456=DIRECTION ( 'NONE',  ( -8.163404592832030268E-17, 1.000000000000000000, -0.000000000000000000 ) ) ;
#6460=EDGE_LOOP ( 'NONE', ( #6234, #1755, #1597, #5873 ) ) ;
#6461=CARTESIAN_POINT ( 'NONE',  ( -824.4888212380172945, 83.64126188030886055, -144.6134169528912423 ) ) ;
#6462=EDGE_CURVE ( 'NONE', #2042, #8251, #6187, .T. ) ;
#6468=AXIS2_PLACEMENT_3D ( 'NONE', #3124, #6896, #1279 ) ;
#6477=ORIENTED_EDGE ( 'NONE', *, *, #10921, .T. ) ;
#6478=CARTESIAN_POINT ( 'NONE',  ( -371.1276969240240646, 59.03915725236748813, -139.2323628767284731 ) ) ;
#6480=VERTEX_POINT ( 'NONE', #4525 ) ;
#6484=DIRECTION ( 'NONE',  ( -8.163404592832030268E-17, 1.000000000000000000, -0.000000000000000000 ) ) ;
#6496=VERTEX_POINT ( 'NONE', #5431 ) ;
#6498=CARTESIAN_POINT ( 'NONE',  ( -371.8248261169420630, 102.8498242185334846, -142.9335005713146529 ) ) ;
#6501=AXIS2_PLACEMENT_3D ( 'NONE', #1860, #2848, #6790 ) ;
#6508=ORIENTED_EDGE ( 'NONE', *, *, #5465, .F. ) ;
#6509=CARTESIAN_POINT ( 'NONE',  ( -379.3580220151804383, 62.32607694421552935, -128.2928256996931111 ) ) ;
#6510=VECTOR ( 'NONE', #8884, 1000.000000000000000 ) ;
#6514=CARTESIAN_POINT ( 'NONE',  ( -119.9999999999999858, -9.213203435596451385, -126.4213562373086575 ) ) ;
#6516=EDGE_CURVE ( 'NONE', #12134, #7292, #2438, .T. ) ;
#6517=FACE_OUTER_BOUND ( 'NONE', #7657, .T. ) ;
#6523=CARTESIAN_POINT ( 'NONE',  ( -821.3235167497176690, 83.01396457509397919, -144.6558853884949087 ) ) ;
#6526=EDGE_LOOP ( 'NONE', ( #5558, #11875 ) ) ;
#6531=APPLICATION_CONTEXT ( 'automotive_design' ) ;
#6532=DIRECTION ( 'NONE',  ( -0.000000000000000000, 1.000000000000000000, -0.000000000000000000 ) ) ;
#6533=CARTESIAN_POINT ( 'NONE',  ( -157.5000000000000000, 139.9999999999999716, -126.4213562373084301 ) ) ;
#6535=CARTESIAN_POINT ( 'NONE',  ( -822.4997677527400128, 73.84243176666221586, -142.9416447491877307 ) ) ;
#6536=VERTEX_POINT ( 'NONE', #8427 ) ;
#6538=CARTESIAN_POINT ( 'NONE',  ( -374.1531042745066316, 71.13268086833227244, -151.9963463910141286 ) ) ;
#6551=CARTESIAN_POINT ( 'NONE',  ( -372.5499461424406604, 101.5496394262485182, -120.1812972028120470 ) ) ;
#6553=EDGE_CURVE ( 'NONE', #11084, #8014, #2853, .T. ) ;
#6556=DIRECTION ( 'NONE',  ( 0.000000000000000000, 1.000000000000000000, -0.000000000000000000 ) ) ;
#6557=ORIENTED_EDGE ( 'NONE', *, *, #5365, .F. ) ;
#6561=CARTESIAN_POINT ( 'NONE',  ( -371.9902837035793368, 102.3136832969389189, -143.7067233690550552 ) ) ;
#6570=FACE_BOUND ( 'NONE', #283, .T. ) ;
#6573=CARTESIAN_POINT ( 'NONE',  ( -374.9207090424860667, 77.70118234822507475, -144.2684479270019153 ) ) ;
#6575=CARTESIAN_POINT ( 'NONE',  ( -383.9497063041636125, 73.38109969229333274, -106.6302449113261872 ) ) ;
#6576=CARTESIAN_POINT ( 'NONE',  ( -119.9999999999999858, -9.213203435596451385, -126.4213562373086575 ) ) ;
#6584=EDGE_LOOP ( 'NONE', ( #4083, #8565, #1931, #2423 ) ) ;
#6587=CARTESIAN_POINT ( 'NONE',  ( -373.3641256762145417, 97.05128668816033155, -100.0945821807713543 ) ) ;
#6593=CARTESIAN_POINT ( 'NONE',  ( -818.8285638327206470, 78.67432280806531253, -104.9592124606049879 ) ) ;
#6608=AXIS2_PLACEMENT_3D ( 'NONE', #9302, #845, #4616 ) ;
#6617=AXIS2_PLACEMENT_3D ( 'NONE', #6434, #10017, #5368 ) ;
#6620=CARTESIAN_POINT ( 'NONE',  ( -370.9145534060840532, 105.5813659013322479, -138.0025389308291608 ) ) ;
#6627=VERTEX_POINT ( 'NONE', #1547 ) ;
#6630=CARTESIAN_POINT ( 'NONE',  ( -374.8135003541144101, 87.17728863486301805, -154.1080623301308208 ) ) ;
#6632=CARTESIAN_POINT ( 'NONE',  ( -384.8761410539145231, 79.01556305096559640, -104.9019531990182088 ) ) ;
#6633=DIRECTION ( 'NONE',  ( -8.163404592832030268E-17, 1.000000000000000000, -0.000000000000000000 ) ) ;
#6638=DIRECTION ( 'NONE',  ( 2.040851148208007875E-17, -1.000000000000000000, -0.000000000000000000 ) ) ;
#6643=CIRCLE ( 'NONE', #314, 7.500000000000007105 ) ;
#6645=CARTESIAN_POINT ( 'NONE',  ( -828.8285638327206470, 78.99577924834029830, -144.4565372401586956 ) ) ;
#6646=PRODUCT_CONTEXT ( 'NONE', #5894, 'mechanical' ) ;
#6647=CARTESIAN_POINT ( 'NONE',  ( -370.4401466759219375, 106.8513018378076964, -134.3428354745942102 ) ) ;
#6648=VERTEX_POINT ( 'NONE', #3511 ) ;
#6649=CARTESIAN_POINT ( 'NONE',  ( -232.4999999999999716, -9.213203435596478030, -126.4213562373078190 ) ) ;
#6651=CARTESIAN_POINT ( 'NONE',  ( -277.5000000000000000, 151.9999999999999716, -126.4213562373076059 ) ) ;
#6652=LINE ( 'NONE', #5356, #6804 ) ;
#6657=FACE_BOUND ( 'NONE', #5, .T. ) ;
#6658=ORIENTED_EDGE ( 'NONE', *, *, #9624, .F. ) ;
#6659=CARTESIAN_POINT ( 'NONE',  ( -374.9651464077482501, 79.71832840036303480, -154.5744145532411267 ) ) ;
#6660=CARTESIAN_POINT ( 'NONE',  ( -373.4738573936541570, 97.83297831077017293, -112.3786037173117194 ) ) ;
#6671=DIRECTION ( 'NONE',  ( -1.000000000000000000, 0.000000000000000000, 0.000000000000000000 ) ) ;
#6676=ORIENTED_EDGE ( 'NONE', *, *, #2393, .T. ) ;
#6677=CARTESIAN_POINT ( 'NONE',  ( -374.5052761646434192, 91.59736101580315903, -142.2979785311488286 ) ) ;
#6679=EDGE_CURVE ( 'NONE', #9394, #1855, #1986, .T. ) ;
#6681=VECTOR ( 'NONE', #6337, 1000.000000000000000 ) ;
#6688=CARTESIAN_POINT ( 'NONE',  ( -374.9845254985059455, 80.12302501620320072, -144.5988415073323665 ) ) ;
#6690=CARTESIAN_POINT ( 'NONE',  ( -384.1592857098779632, 74.28227529662643747, -106.2268997244850652 ) ) ;
#6697=ADVANCED_FACE ( 'NONE', ( #4710 ), #4820, .F. ) ;
#6700=CIRCLE ( 'NONE', #2955, 57.99999999999999289 ) ;
#6703=CARTESIAN_POINT ( 'NONE',  ( -383.7561884827940730, 72.61679055868643218, -107.0088101474849793 ) ) ;
#6707=CARTESIAN_POINT ( 'NONE',  ( -372.2669691774863736, 101.3813217465900323, -104.4136360144974134 ) ) ;
#6711=CARTESIAN_POINT ( 'NONE',  ( -187.5000000000000000, 151.9999999999999716, -126.4213562373082453 ) ) ;
#6714=CARTESIAN_POINT ( 'NONE',  ( 35.00000000000000000, 139.9999999999999716, -89.68077099980384048 ) ) ;
#6718=CARTESIAN_POINT ( 'NONE',  ( -381.2985570915043922, 98.03646409573219955, -112.7250802902767219 ) ) ;
#6724=ORIENTED_EDGE ( 'NONE', *, *, #6451, .T. ) ;
#6725=DIRECTION ( 'NONE',  ( -1.000000000000000000, 0.000000000000000000, 0.000000000000000000 ) ) ;
#6734=PRODUCT ( 'Long Manual Ratchet Lever Handle', 'Long Manual Ratchet Lever Handle', '', ( #6646 ) ) ;
#6744=CARTESIAN_POINT ( 'NONE',  ( -374.4862286338727699, 72.16765808346663391, -142.2089878380306800 ) ) ;
#6745=CARTESIAN_POINT ( 'NONE',  ( -59.99999999999998579, 24.00000000000001421, -126.4213562373090696 ) ) ;
#6746=CARTESIAN_POINT ( 'NONE',  ( -374.7871828591273697, 75.45048456915552038, -105.7389799933290817 ) ) ;
#6748=DIRECTION ( 'NONE',  ( 1.000000000000000000, -0.000000000000000000, -0.000000000000000000 ) ) ;
#6773=LINE ( 'NONE', #3999, #1084 ) ;
#6774=ORIENTED_EDGE ( 'NONE', *, *, #708, .T. ) ;
#6775=CARTESIAN_POINT ( 'NONE',  ( 1.959217102279688941E-15, 139.9999999999999716, -126.4213562373094959 ) ) ;
#6776=CARTESIAN_POINT ( 'NONE',  ( -384.5214733245267666, 87.83340981944037651, -105.5475429248750032 ) ) ;
#6778=EDGE_LOOP ( 'NONE', ( #12021, #4214 ) ) ;
#6780=EDGE_CURVE ( 'NONE', #7586, #6370, #6012, .T. ) ;
#6781=CARTESIAN_POINT ( 'NONE',  ( -210.0000000000000000, -9.213203435596478030, -126.4213562373080180 ) ) ;
#6787=CARTESIAN_POINT ( 'NONE',  ( -818.9856806503953521, 79.95950042231982025, -104.7825536331197043 ) ) ;
#6790=DIRECTION ( 'NONE',  ( -1.000000000000000000, 0.000000000000000000, 0.000000000000000000 ) ) ;
#6791=DIRECTION ( 'NONE',  ( -8.163404592832030268E-17, 1.000000000000000000, -0.000000000000000000 ) ) ;
#6793=EDGE_LOOP ( 'NONE', ( #3710, #1617 ) ) ;
#6795=AXIS2_PLACEMENT_3D ( 'NONE', #1123, #7664, #10380 ) ;
#6801=ORIENTED_EDGE ( 'NONE', *, *, #342, .F. ) ;
#6803=CARTESIAN_POINT ( 'NONE',  ( -127.4999999999999716, 24.00000000000001421, -126.4213562373086575 ) ) ;
#6804=VECTOR ( 'NONE', #11920, 1000.000000000000000 ) ;
#6805=FACE_OUTER_BOUND ( 'NONE', #7494, .T. ) ;
#6809=ORIENTED_EDGE ( 'NONE', *, *, #2319, .T. ) ;
#6810=CARTESIAN_POINT ( 'NONE',  ( -374.2117181976924485, 71.51684740197940471, -152.1890516768436612 ) ) ;
#6812=CARTESIAN_POINT ( 'NONE',  ( -374.1390116440427960, 69.71711930496753951, -108.8128785988674849 ) ) ;
#6813=EDGE_LOOP ( 'NONE', ( #10508, #11047, #10675, #8494 ) ) ;
#6817=EDGE_CURVE ( 'NONE', #6480, #11140, #11433, .T. ) ;
#6820=EDGE_CURVE ( 'NONE', #8735, #8014, #3026, .T. ) ;
#6822=FACE_OUTER_BOUND ( 'NONE', #8422, .T. ) ;
#6827=CARTESIAN_POINT ( 'NONE',  ( -384.7926048166160058, 85.88261479689718669, -105.0522379990735544 ) ) ;
#6829=EDGE_LOOP ( 'NONE', ( #7429, #5435, #4946, #12144, #179, #5657, #6724, #2834, #9003, #3940 ) ) ;
#6832=CARTESIAN_POINT ( 'NONE',  ( -305.0000000000000568, 12.00000000000001066, -89.68077099980384048 ) ) ;
#6833=CYLINDRICAL_SURFACE ( 'NONE', #12142, 7.500000000000007105 ) ;
#6834=PRODUCT_DEFINITION_FORMATION_WITH_SPECIFIED_SOURCE ( 'ANY', '', #6734, .NOT_KNOWN. ) ;
#6842=CARTESIAN_POINT ( 'NONE',  ( -384.6205072238515186, 87.19846374239256193, -105.3653610531364251 ) ) ;
#6844=ORIENTED_EDGE ( 'NONE', *, *, #10817, .T. ) ;
#6845=DIRECTION ( 'NONE',  ( 3.061276722312011504E-17, -1.000000000000000000, 0.000000000000000000 ) ) ;
#6848=ORIENTED_EDGE ( 'NONE', *, *, #9702, .T. ) ;
#6852=ORIENTED_EDGE ( 'NONE', *, *, #1344, .F. ) ;
#6854=AXIS2_PLACEMENT_3D ( 'NONE', #8674, #3964, #11386 ) ;
#6865=CIRCLE ( 'NONE', #11214, 7.500000000000007105 ) ;
#6868=EDGE_LOOP ( 'NONE', ( #7680, #9790 ) ) ;
#6876=CARTESIAN_POINT ( 'NONE',  ( -381.9362497754162291, 67.37496909217159669, -111.0233266882457173 ) ) ;
#6878=VECTOR ( 'NONE', #7239, 1000.000000000000000 ) ;
#6880=DIRECTION ( 'NONE',  ( -1.000000000000000000, 0.000000000000000000, 0.000000000000000000 ) ) ;
#6885=CARTESIAN_POINT ( 'NONE',  ( -382.3424684326698184, 95.66281168084425701, -110.0297798447839881 ) ) ;
#6887=EDGE_LOOP ( 'NONE', ( #9537, #3861, #6809, #2934 ) ) ;
#6896=DIRECTION ( 'NONE',  ( 2.040851148208007875E-17, -1.000000000000000000, -0.000000000000000000 ) ) ;
#6900=EDGE_LOOP ( 'NONE', ( #1108, #9962, #11715, #7309 ) ) ;
#6911=CARTESIAN_POINT ( 'NONE',  ( -822.2163178171774689, 83.41010758653600021, -104.7304854148471804 ) ) ;
#6916=CARTESIAN_POINT ( 'NONE',  ( 1.240837498110468453E-14, 12.00000000000001776, -126.4213562373094959 ) ) ;
#6917=FACE_OUTER_BOUND ( 'NONE', #143, .T. ) ;
#6921=EDGE_CURVE ( 'NONE', #8281, #9710, #2655, .T. ) ;
#6934=CARTESIAN_POINT ( 'NONE',  ( -82.49999999999997158, 12.00000000000001421, -126.4213562373088564 ) ) ;
#6935=CARTESIAN_POINT ( 'NONE',  ( -305.0000000000000568, 139.9999999999999716, -89.68077099980384048 ) ) ;
#6944=ORIENTED_EDGE ( 'NONE', *, *, #10601, .F. ) ;
#6950=VERTEX_POINT ( 'NONE', #10970 ) ;
#6953=CARTESIAN_POINT ( 'NONE',  ( -270.0000000000000000, 12.00000000000001066, -126.4213562373076059 ) ) ;
#6958=CARTESIAN_POINT ( 'NONE',  ( -240.0000000000000000, 12.00000000000001066, -126.4213562373078190 ) ) ;
#6959=AXIS2_PLACEMENT_3D ( 'NONE', #9905, #9786, #1439 ) ;
#6965=CARTESIAN_POINT ( 'NONE',  ( -60.00000000000000000, 139.9999999999999716, -126.4213562373090696 ) ) ;
#6969=EDGE_CURVE ( 'NONE', #4621, #7284, #8397, .T. ) ;
#6973=CARTESIAN_POINT ( 'NONE',  ( -370.8011028251392531, 105.8825848193712460, -112.1920252379657796 ) ) ;
#6976=DIRECTION ( 'NONE',  ( -8.163404592832030268E-17, 1.000000000000000000, -0.000000000000000000 ) ) ;
#6980=CARTESIAN_POINT ( 'NONE',  ( -374.9097930543319421, 78.37721037988610817, -94.95651375212828782 ) ) ;
#6981=AXIS2_PLACEMENT_3D ( 'NONE', #369, #4150, #2356 ) ;
#6984=CARTESIAN_POINT ( 'NONE',  ( -380.5583952655373992, 64.47352604413475774, -134.3328398924245448 ) ) ;
#6989=CARTESIAN_POINT ( 'NONE',  ( 0.000000000000000000, 12.00000000000001776, -124.6807709998038405 ) ) ;
#6993=DIRECTION ( 'NONE',  ( 1.000000000000000000, 0.000000000000000000, 0.000000000000000000 ) ) ;
#7016=CARTESIAN_POINT ( 'NONE',  ( -925.0000000000000000, 81.99999999999988631, -124.6807709998038405 ) ) ;
#7017=EDGE_LOOP ( 'NONE', ( #8099, #4002, #2364, #12136 ) ) ;
#7019=CARTESIAN_POINT ( 'NONE',  ( -370.5475656004942380, 57.43166175920264038, -114.0709556960625406 ) ) ;
#7026=DIRECTION ( 'NONE',  ( -1.000000000000000000, 0.000000000000000000, 0.000000000000000000 ) ) ;
#7028=DIRECTION ( 'NONE',  ( 2.040851148208007875E-17, -1.000000000000000000, -0.000000000000000000 ) ) ;
#7033=CIRCLE ( 'NONE', #1715, 7.500000000000007105 ) ;
#7035=VERTEX_POINT ( 'NONE', #11961 ) ;
#7038=EDGE_CURVE ( 'NONE', #1615, #1810, #2264, .T. ) ;
#7040=CARTESIAN_POINT ( 'NONE',  ( -374.1184086109046802, 70.90605591669974217, -97.47965622763319971 ) ) ;
#7044=CARTESIAN_POINT ( 'NONE',  ( -380.0144971365231754, 63.46555453814624315, -132.2185027065989686 ) ) ;
#7045=CARTESIAN_POINT ( 'NONE',  ( -372.1715096098437243, 101.7023887269710229, -144.5189483497782987 ) ) ;
#7046=CARTESIAN_POINT ( 'NONE',  ( -180.0000000000000000, 12.00000000000001421, -126.4213562373082453 ) ) ;
#7057=DIRECTION ( 'NONE',  ( 0.000000000000000000, 1.000000000000000000, -0.000000000000000000 ) ) ;
#7059=ORIENTED_EDGE ( 'NONE', *, *, #12118, .T. ) ;
#7066=VECTOR ( 'NONE', #10864, 1000.000000000000000 ) ;
#7068=EDGE_CURVE ( 'NONE', #818, #10791, #11779, .T. ) ;
#7076=DIRECTION ( 'NONE',  ( -1.000000000000000000, 0.000000000000000000, 0.000000000000000000 ) ) ;
#7080=CIRCLE ( 'NONE', #568, 7.500000000000020428 ) ;
#7082=ORIENTED_EDGE ( 'NONE', *, *, #10228, .T. ) ;
#7091=AXIS2_PLACEMENT_3D ( 'NONE', #3825, #741, #4519 ) ;
#7093=CARTESIAN_POINT ( 'NONE',  ( -828.6703486388499869, 79.96407734986385663, -104.7820573548426069 ) ) ;
#7095=CIRCLE ( 'NONE', #5916, 7.500000000000007105 ) ;
#7097=FACE_OUTER_BOUND ( 'NONE', #4169, .T. ) ;
#7101=DIRECTION ( 'NONE',  ( -0.000000000000000000, -0.000000000000000000, -1.000000000000000000 ) ) ;
#7102=CARTESIAN_POINT ( 'NONE',  ( -375.0000000000000568, 82.00000000000093792, -94.68077099980381206 ) ) ;
#7103=CARTESIAN_POINT ( 'NONE',  ( -374.7780441258248061, 76.25198850915256799, -95.36283402834658318 ) ) ;
#7106=EDGE_LOOP ( 'NONE', ( #10294, #10262, #5913, #7390 ) ) ;
#7107=CARTESIAN_POINT ( 'NONE',  ( -383.0048299740013249, 70.12786572434940524, -140.8172186891583237 ) ) ;
#7110=CARTESIAN_POINT ( 'NONE',  ( -370.7831763668500571, 105.9365648485286471, -137.0819547014295097 ) ) ;
#7116=VERTEX_POINT ( 'NONE', #204 ) ;
#7124=ORIENTED_EDGE ( 'NONE', *, *, #7068, .F. ) ;
#7125=CYLINDRICAL_SURFACE ( 'NONE', #5364, 7.500000000000007994 ) ;
#7129=EDGE_CURVE ( 'NONE', #2078, #3022, #3238, .T. ) ;
#7134=CARTESIAN_POINT ( 'NONE',  ( 0.000000000000000000, 139.9999999999999716, -124.6807709998038405 ) ) ;
#7135=CARTESIAN_POINT ( 'NONE',  ( -925.0000000000000000, 61.99999999999980815, -124.6807709998038405 ) ) ;
#7136=CARTESIAN_POINT ( 'NONE',  ( -374.9726451943776055, 84.25168756434180750, -94.76384896039375860 ) ) ;
#7139=CARTESIAN_POINT ( 'NONE',  ( -379.9115039592767857, 63.28126683224602544, -117.6075586578124046 ) ) ;
#7140=AXIS2_PLACEMENT_3D ( 'NONE', #11175, #8275, #10916 ) ;
#7147=CARTESIAN_POINT ( 'NONE',  ( 9.796085511398436814E-16, 152.0000000000000000, -126.4213562373094959 ) ) ;
#7151=CIRCLE ( 'NONE', #8736, 20.00000000000008882 ) ;
#7153=DIRECTION ( 'NONE',  ( -0.000000000000000000, -0.000000000000000000, -1.000000000000000000 ) ) ;
#7154=CARTESIAN_POINT ( 'NONE',  ( -819.4840074578143003, 76.17856360854463560, -143.8168744253322870 ) ) ;
#7157=CARTESIAN_POINT ( 'NONE',  ( 0.000000000000000000, 24.00000000000001776, -124.6807709998038405 ) ) ;
#7160=EDGE_LOOP ( 'NONE', ( #263, #4905, #1027, #4930, #2466 ) ) ;
#7164=LINE ( 'NONE', #4324, #7066 ) ;
#7165=CARTESIAN_POINT ( 'NONE',  ( -217.5000000000000000, 12.00000000000001421, -126.4213562373080180 ) ) ;
#7168=AXIS2_PLACEMENT_3D ( 'NONE', #10685, #5989, #9758 ) ;
#7178=DIRECTION ( 'NONE',  ( -8.163404592832030268E-17, 1.000000000000000000, -0.000000000000000000 ) ) ;
#7182=CARTESIAN_POINT ( 'NONE',  ( -120.0000000000000000, 152.0000000000000000, -126.4213562373086575 ) ) ;
#7183=AXIS2_PLACEMENT_3D ( 'NONE', #3429, #11110, #10054 ) ;
#7187=CARTESIAN_POINT ( 'NONE',  ( -379.7921418149325063, 63.07164944986214294, -118.2218589047913468 ) ) ;
#7188=CARTESIAN_POINT ( 'NONE',  ( -379.4171904840047205, 101.5744813863694134, -120.5347007855791617 ) ) ;
#7192=CIRCLE ( 'NONE', #10158, 7.500000000000007105 ) ;
#7198=FACE_OUTER_BOUND ( 'NONE', #6584, .T. ) ;
#7200=VECTOR ( 'NONE', #2977, 1000.000000000000000 ) ;
#7214=EDGE_CURVE ( 'NONE', #609, #5232, #7192, .T. ) ;
#7216=CARTESIAN_POINT ( 'NONE',  ( -823.1581254408797577, 73.70809864670201250, -142.8810402703304021 ) ) ;
#7225=CARTESIAN_POINT ( 'NONE',  ( 0.000000000000000000, 81.99999999999995737, -159.6807709998038547 ) ) ;
#7229=ORIENTED_EDGE ( 'NONE', *, *, #10550, .T. ) ;
#7234=CARTESIAN_POINT ( 'NONE',  ( -385.0037317092140370, 81.69534135820630638, -144.6874058649623862 ) ) ;
#7239=DIRECTION ( 'NONE',  ( -8.163404592832030268E-17, 1.000000000000000000, -0.000000000000000000 ) ) ;
#7240=CYLINDRICAL_SURFACE ( 'NONE', #9231, 7.500000000000007105 ) ;
#7250=AXIS2_PLACEMENT_3D ( 'NONE', #9366, #6456, #6393 ) ;
#7251=CARTESIAN_POINT ( 'NONE',  ( -370.2091804001356081, 56.54852862931996071, -132.0405513051967716 ) ) ;
#7261=CARTESIAN_POINT ( 'NONE',  ( -305.0000000000000568, 24.00000000000000711, -159.6807709998038547 ) ) ;
#7264=CIRCLE ( 'NONE', #1942, 7.500000000000007105 ) ;
#7273=AXIS2_PLACEMENT_3D ( 'NONE', #1099, #9553, #5721 ) ;
#7284=VERTEX_POINT ( 'NONE', #2193 ) ;
#7289=CARTESIAN_POINT ( 'NONE',  ( -90.00000000000000000, 152.0000000000000000, -126.4213562373088564 ) ) ;
#7292=VERTEX_POINT ( 'NONE', #8860 ) ;
#7294=VECTOR ( 'NONE', #11792, 1000.000000000000000 ) ;
#7300=CARTESIAN_POINT ( 'NONE',  ( -372.6517233435575918, 101.1862970994316697, -130.5563829983385347 ) ) ;
#7309=ORIENTED_EDGE ( 'NONE', *, *, #1083, .T. ) ;
#7317=CARTESIAN_POINT ( 'NONE',  ( -369.9778043404595564, 55.96332071781321105, -128.6253823055326961 ) ) ;
#7319=VERTEX_POINT ( 'NONE', #9281 ) ;
#7328=DIRECTION ( 'NONE',  ( 2.040851148208007875E-17, -1.000000000000000000, -0.000000000000000000 ) ) ;
#7329=CARTESIAN_POINT ( 'NONE',  ( -374.0809930161825605, 70.68769334614165700, -97.60498186712243296 ) ) ;
#7330=ORIENTED_EDGE ( 'NONE', *, *, #9624, .T. ) ;
#7331=CARTESIAN_POINT ( 'NONE',  ( -823.1761409384598664, 83.64233031452180001, -144.6133277457489612 ) ) ;
#7333=DIRECTION ( 'NONE',  ( -1.000000000000000000, 0.000000000000000000, 0.000000000000000000 ) ) ;
#7335=DIRECTION ( 'NONE',  ( 0.000000000000000000, 0.000000000000000000, 1.000000000000000000 ) ) ;
#7338=CARTESIAN_POINT ( 'NONE',  ( -827.8145948178535036, 75.63860347950554797, -143.6442145102265329 ) ) ;
#7342=CARTESIAN_POINT ( 'NONE',  ( -370.7999735434212880, 58.11281947991218999, -137.1733638493476519 ) ) ;
#7346=CARTESIAN_POINT ( 'NONE',  ( -30.00000000000000000, 152.0000000000000000, -126.4213562373092685 ) ) ;
#7347=LINE ( 'NONE', #6352, #8470 ) ;
#7348=CARTESIAN_POINT ( 'NONE',  ( -373.0722496536144490, 65.67588619885601986, -101.1744612802395125 ) ) ;
#7355=CYLINDRICAL_SURFACE ( 'NONE', #7091, 20.00000000000004619 ) ;
#7358=CARTESIAN_POINT ( 'NONE',  ( -369.9085427289805921, 108.2084335843136387, -126.6389740589983433 ) ) ;
#7363=ORIENTED_EDGE ( 'NONE', *, *, #2285, .T. ) ;
#7365=DIRECTION ( 'NONE',  ( -1.000000000000000000, 0.000000000000000000, 0.000000000000000000 ) ) ;
#7370=VERTEX_POINT ( 'NONE', #1707 ) ;
#7375=VERTEX_POINT ( 'NONE', #9243 ) ;
#7376=ADVANCED_FACE ( 'NONE', ( #359 ), #2283, .F. ) ;
#7377=CARTESIAN_POINT ( 'NONE',  ( -373.1538797604212050, 64.77014134620993957, -134.9108730226440969 ) ) ;
#7379=CARTESIAN_POINT ( 'NONE',  ( -232.4999999999999716, 12.00000000000001066, -126.4213562373078190 ) ) ;
#7384=DIRECTION ( 'NONE',  ( -8.163404592832030268E-17, 1.000000000000000000, -0.000000000000000000 ) ) ;
#7390=ORIENTED_EDGE ( 'NONE', *, *, #8880, .T. ) ;
#7392=CARTESIAN_POINT ( 'NONE',  ( -823.5011194091124480, 83.67446401253047839, -144.6105519893419000 ) ) ;
#7394=CIRCLE ( 'NONE', #11343, 7.500000000000007105 ) ;
#7395=CARTESIAN_POINT ( 'NONE',  ( -369.8899886004867881, 108.2543221321664930, -124.8540024292112065 ) ) ;
#7405=CARTESIAN_POINT ( 'NONE',  ( -827.1548796934557686, 74.92718183615713201, -143.3900093790822439 ) ) ;
#7408=CARTESIAN_POINT ( 'NONE',  ( -369.9667548185103669, 55.93616024285574895, -121.0690321629715669 ) ) ;
#7413=DIRECTION ( 'NONE',  ( 2.040851148208007875E-17, -1.000000000000000000, -0.000000000000000000 ) ) ;
#7414=CARTESIAN_POINT ( 'NONE',  ( -371.0944895696485446, 58.94320524275045159, -110.3215891064999994 ) ) ;
#7422=ADVANCED_FACE ( 'NONE', ( #11077, #8114 ), #180, .T. ) ;
#7425=CARTESIAN_POINT ( 'NONE',  ( -262.5000000000000000, -9.213203435596478030, -126.4213562373076059 ) ) ;
#7429=ORIENTED_EDGE ( 'NONE', *, *, #4516, .T. ) ;
#7433=CARTESIAN_POINT ( 'NONE',  ( -374.1032283779920817, 69.49316288506409478, -140.3724387714157444 ) ) ;
#7436=AXIS2_PLACEMENT_3D ( 'NONE', #1888, #9102, #7333 ) ;
#7440=EDGE_CURVE ( 'NONE', #9588, #8369, #3, .T. ) ;
#7443=CIRCLE ( 'NONE', #5260, 7.499999999999992895 ) ;
#7446=CARTESIAN_POINT ( 'NONE',  ( -379.1619848709565304, 102.0000000000000142, -125.7938822953540381 ) ) ;
#7448=CARTESIAN_POINT ( 'NONE',  ( -818.9871366297743407, 79.96561131120978416, -144.5796535119514488 ) ) ;
#7460=CARTESIAN_POINT ( 'NONE',  ( -210.0000000000000000, 151.9999999999999716, -126.4213562373080180 ) ) ;
#7461=CARTESIAN_POINT ( 'NONE',  ( 0.000000000000000000, 152.0000000000000000, -124.6807709998038405 ) ) ;
#7464=CARTESIAN_POINT ( 'NONE',  ( -819.0854767918228845, 77.05939038872129743, -105.2981374327913358 ) ) ;
#7466=CARTESIAN_POINT ( 'NONE',  ( -821.2963138009649811, 74.35985007445651718, -143.1641509997125183 ) ) ;
#7467=VECTOR ( 'NONE', #6748, 1000.000000000000000 ) ;
#7469=CARTESIAN_POINT ( 'NONE',  ( -373.9059702089900270, 69.66321476674123403, -151.1683612898431477 ) ) ;
#7470=CARTESIAN_POINT ( 'NONE',  ( -374.4452484659049105, 92.10134583476683190, -107.3453501722017052 ) ) ;
#7473=EDGE_CURVE ( 'NONE', #8380, #3503, #3058, .T. ) ;
#7480=LINE ( 'NONE', #11369, #787 ) ;
#7483=CARTESIAN_POINT ( 'NONE',  ( -379.6804543574866670, 101.1236513765119724, -118.8160366733158639 ) ) ;
#7484=AXIS2_PLACEMENT_3D ( 'NONE', #6781, #10497, #4129 ) ;
#7490=CARTESIAN_POINT ( 'NONE',  ( -374.5977935108010684, 90.76354315037471565, -142.7312558896330756 ) ) ;
#7494=EDGE_LOOP ( 'NONE', ( #9053, #11774, #6774, #4293 ) ) ;
#7498=VERTEX_POINT ( 'NONE', #6803 ) ;
#7499=CARTESIAN_POINT ( 'NONE',  ( -382.3282078984223631, 68.32957519679821701, -139.2830325097624495 ) ) ;
#7501=CIRCLE ( 'NONE', #4339, 7.500000000000007105 ) ;
#7515=DIRECTION ( 'NONE',  ( 0.000000000000000000, 0.000000000000000000, 1.000000000000000000 ) ) ;
#7523=CARTESIAN_POINT ( 'NONE',  ( -825.4664863774313517, 73.94730815836251736, -106.3734765325340561 ) ) ;
#7527=ORIENTED_EDGE ( 'NONE', *, *, #10928, .T. ) ;
#7529=CARTESIAN_POINT ( 'NONE',  ( -380.9366354222731843, 98.78228965653478610, -113.7968190044388450 ) ) ;
#7539=CARTESIAN_POINT ( 'NONE',  ( -59.99999999999998579, -9.213203435596451385, -126.4213562373090696 ) ) ;
#7547=ORIENTED_EDGE ( 'NONE', *, *, #7038, .F. ) ;
#7557=CARTESIAN_POINT ( 'NONE',  ( -384.6392999096204335, 76.78897796811929766, -144.0344280892469158 ) ) ;
#7559=CARTESIAN_POINT ( 'NONE',  ( -374.7455030271728447, 74.89167502208620419, -105.9368347594480753 ) ) ;
#7560=DIRECTION ( 'NONE',  ( 3.061276722312011504E-17, -1.000000000000000000, 0.000000000000000000 ) ) ;
#7569=VERTEX_POINT ( 'NONE', #2190 ) ;
#7574=ORIENTED_EDGE ( 'NONE', *, *, #2079, .T. ) ;
#7581=DIRECTION ( 'NONE',  ( 2.040851148208007875E-17, -1.000000000000000000, -0.000000000000000000 ) ) ;
#7586=VERTEX_POINT ( 'NONE', #9230 ) ;
#7588=CARTESIAN_POINT ( 'NONE',  ( -384.4682197693251169, 88.14714501232053578, -105.6460668681738753 ) ) ;
#7591=ADVANCED_FACE ( 'NONE', ( #6517 ), #11153, .F. ) ;
#7595=EDGE_CURVE ( 'NONE', #4244, #10520, #3246, .T. ) ;
#7603=CARTESIAN_POINT ( 'NONE',  ( -372.6969993560938406, 101.0120954562736415, -118.4175876187035215 ) ) ;
#7611=CARTESIAN_POINT ( 'NONE',  ( -371.3527037074148325, 104.3051788345223230, -140.5275824910885660 ) ) ;
#7615=EDGE_LOOP ( 'NONE', ( #6356, #2887, #9201, #3740 ) ) ;
#7621=CARTESIAN_POINT ( 'NONE',  ( -374.9952863086498951, 80.93532140996973112, -144.6556666394729120 ) ) ;
#7623=CARTESIAN_POINT ( 'NONE',  ( -384.9453241936137147, 80.00116030919089383, -104.7781441965376814 ) ) ;
#7624=CARTESIAN_POINT ( 'NONE',  ( -119.9999999999999858, 24.00000000000001421, -126.4213562373086575 ) ) ;
#7626=ORIENTED_EDGE ( 'NONE', *, *, #8722, .F. ) ;
#7629=LINE ( 'NONE', #960, #2303 ) ;
#7634=AXIS2_PLACEMENT_3D ( 'NONE', #3554, #8149, #2515 ) ;
#7635=CARTESIAN_POINT ( 'NONE',  ( -82.49999999999998579, 139.9999999999999716, -126.4213562373088564 ) ) ;
#7642=DIRECTION ( 'NONE',  ( -1.000000000000000000, 0.000000000000000000, 0.000000000000000000 ) ) ;
#7648=CARTESIAN_POINT ( 'NONE',  ( -374.5346922981962052, 90.06812782866809641, -96.12871480239243738 ) ) ;
#7657=EDGE_LOOP ( 'NONE', ( #2544, #1974, #7943, #8751 ) ) ;
#7660=FACE_OUTER_BOUND ( 'NONE', #9255, .T. ) ;
#7664=DIRECTION ( 'NONE',  ( -8.163404592832031500E-17, 1.000000000000000000, 0.000000000000000000 ) ) ;
#7671=ORIENTED_EDGE ( 'NONE', *, *, #9780, .F. ) ;
#7678=FACE_BOUND ( 'NONE', #316, .T. ) ;
#7680=ORIENTED_EDGE ( 'NONE', *, *, #2393, .F. ) ;
#7682=CARTESIAN_POINT ( 'NONE',  ( -374.9895210541299662, 83.62267570606550748, -144.6251211967523034 ) ) ;
#7684=CARTESIAN_POINT ( 'NONE',  ( -374.4827113483042922, 72.13547865759302624, -107.1640604315173988 ) ) ;
#7693=EDGE_CURVE ( 'NONE', #7116, #5834, #5451, .T. ) ;
#7695=CARTESIAN_POINT ( 'NONE',  ( -383.4612065782806098, 92.42287728680335590, -107.6015166696609668 ) ) ;
#7697=VERTEX_POINT ( 'NONE', #1762 ) ;
#7700=EDGE_LOOP ( 'NONE', ( #1712, #11876, #5961, #1447 ) ) ;
#7703=CARTESIAN_POINT ( 'NONE',  ( -157.5000000000000000, 12.00000000000001421, -126.4213562373084301 ) ) ;
#7705=FACE_BOUND ( 'NONE', #11908, .T. ) ;
#7718=CARTESIAN_POINT ( 'NONE',  ( -371.0721991683506644, 105.1220130550264997, -110.4447908282102446 ) ) ;
#7724=DIRECTION ( 'NONE',  ( -8.163404592832031500E-17, 1.000000000000000000, 0.000000000000000000 ) ) ;
#7732=CARTESIAN_POINT ( 'NONE',  ( -381.3400711680802146, 97.95158805382058631, -136.7590353381492889 ) ) ;
#7735=AXIS2_PLACEMENT_3D ( 'NONE', #5354, #3557, #1535 ) ;
#7737=CARTESIAN_POINT ( 'NONE',  ( -374.7451988284479398, 88.02670150610194355, -153.8963740139208483 ) ) ;
#7739=CARTESIAN_POINT ( 'NONE',  ( -383.5775985103214794, 71.91734269553219860, -107.3587914639481653 ) ) ;
#7745=VERTEX_POINT ( 'NONE', #9033 ) ;
#7746=CARTESIAN_POINT ( 'NONE',  ( -150.0000000000000000, 12.00000000000001421, -126.4213562373084301 ) ) ;
#7747=EDGE_CURVE ( 'NONE', #2602, #9984, #8977, .T. ) ;
#7765=CARTESIAN_POINT ( 'NONE',  ( -232.4999999999999716, 24.00000000000000711, -126.4213562373078190 ) ) ;
#7767=VERTEX_POINT ( 'NONE', #6203 ) ;
#7768=CARTESIAN_POINT ( 'NONE',  ( -374.5759732026825759, 74.23177511559134700, -153.3650736963693078 ) ) ;
#7776=AXIS2_PLACEMENT_3D ( 'NONE', #164, #1914, #9453 ) ;
#7777=VECTOR ( 'NONE', #11201, 1000.000000000000000 ) ;
#7781=CARTESIAN_POINT ( 'NONE',  ( -820.7717470982031500, 82.64484858469192829, -104.6903222377186893 ) ) ;
#7784=CARTESIAN_POINT ( 'NONE',  ( -380.6764949106236600, 99.29952767699337812, -114.6234865369922034 ) ) ;
#7797=VERTEX_POINT ( 'NONE', #8181 ) ;
#7801=FACE_BOUND ( 'NONE', #2192, .T. ) ;
#7803=CARTESIAN_POINT ( 'NONE',  ( -37.49999999999999289, 12.00000000000001776, -126.4213562373092685 ) ) ;
#7805=CARTESIAN_POINT ( 'NONE',  ( -374.0261869715998273, 70.33727264991432548, -151.5753310962235503 ) ) ;
#7807=ORIENTED_EDGE ( 'NONE', *, *, #2610, .T. ) ;
#7810=ORIENTED_EDGE ( 'NONE', *, *, #3087, .T. ) ;
#7811=ORIENTED_EDGE ( 'NONE', *, *, #9267, .T. ) ;
#7816=ORIENTED_EDGE ( 'NONE', *, *, #860, .T. ) ;
#7818=DIRECTION ( 'NONE',  ( -1.000000000000000000, 0.000000000000000000, 0.000000000000000000 ) ) ;
#7825=CARTESIAN_POINT ( 'NONE',  ( -89.99999999999998579, 24.00000000000001421, -126.4213562373088564 ) ) ;
#7834=ADVANCED_FACE ( 'NONE', ( #4608 ), #1017, .F. ) ;
#7842=EDGE_CURVE ( 'NONE', #11231, #1969, #1080, .T. ) ;
#7861=CARTESIAN_POINT ( 'NONE',  ( -7.499999999999994671, -9.213203435596451385, -126.4213562373094959 ) ) ;
#7864=CARTESIAN_POINT ( 'NONE',  ( -384.7284696814416520, 86.42946640087690469, -144.1932104012986429 ) ) ;
#7868=CARTESIAN_POINT ( 'NONE',  ( -374.8244134398003098, 87.00545050162834571, -154.1417378514361758 ) ) ;
#7869=LINE ( 'NONE', #373, #1867 ) ;
#7871=B_SPLINE_CURVE_WITH_KNOTS ( 'NONE', 3,
 ( #3673, #7446, #2756, #11229, #1830, #4902 ),
 .UNSPECIFIED., .F., .F.,
 ( 4, 2, 4 ),
 ( 0.000000000000000000, 0.003279474516629658862, 0.006558949033259317725 ),
 .UNSPECIFIED. ) ;
#7880=CARTESIAN_POINT ( 'NONE',  ( -210.0000000000000000, -9.213203435596478030, -126.4213562373080180 ) ) ;
#7891=DIRECTION ( 'NONE',  ( 1.000000000000000000, 0.000000000000000000, 0.000000000000000000 ) ) ;
#7893=CIRCLE ( 'NONE', #10454, 7.500000000000007105 ) ;
#7899=AXIS2_PLACEMENT_3D ( 'NONE', #6714, #9500, #2090 ) ;
#7906=ADVANCED_FACE ( 'NONE', ( #12206 ), #8503, .F. ) ;
#7911=CARTESIAN_POINT ( 'NONE',  ( -379.7921418149325063, 63.07164944986214294, -118.2218589047913611 ) ) ;
#7912=CARTESIAN_POINT ( 'NONE',  ( -380.0568384841039915, 100.4584982090781295, -116.9531293578063327 ) ) ;
#7915=ORIENTED_EDGE ( 'NONE', *, *, #7068, .T. ) ;
#7920=CARTESIAN_POINT ( 'NONE',  ( -305.0000000000000568, 81.99999999999995737, -89.68077099980384048 ) ) ;
#7921=ORIENTED_EDGE ( 'NONE', *, *, #6377, .T. ) ;
#7922=EDGE_CURVE ( 'NONE', #9588, #7116, #4104, .T. ) ;
#7924=CARTESIAN_POINT ( 'NONE',  ( -381.8376525299339619, 67.14791246521063783, -138.0876920893665272 ) ) ;
#7929=FILL_AREA_STYLE_COLOUR ( '', #8254 ) ;
#7937=ORIENTED_EDGE ( 'NONE', *, *, #1560, .T. ) ;
#7940=ORIENTED_EDGE ( 'NONE', *, *, #4216, .T. ) ;
#7943=ORIENTED_EDGE ( 'NONE', *, *, #6229, .F. ) ;
#7945=CARTESIAN_POINT ( 'NONE',  ( -67.49999999999998579, 24.00000000000001421, -126.4213562373090696 ) ) ;
#7955=DIRECTION ( 'NONE',  ( 1.000000000000000000, 0.000000000000000000, 0.000000000000000000 ) ) ;
#7958=ORIENTED_EDGE ( 'NONE', *, *, #6679, .T. ) ;
#7964=DIRECTION ( 'NONE',  ( -8.163404592832031500E-17, 1.000000000000000000, 0.000000000000000000 ) ) ;
#7965=CARTESIAN_POINT ( 'NONE',  ( -240.0000000000000000, -9.213203435596478030, -126.4213562373078190 ) ) ;
#7968=CARTESIAN_POINT ( 'NONE',  ( -828.8285638327203060, 78.83536470144997566, -104.9320557148177926 ) ) ;
#7969=CARTESIAN_POINT ( 'NONE',  ( -112.4999999999999858, 139.9999999999999716, -126.4213562373086575 ) ) ;
#7973=FACE_BOUND ( 'NONE', #5380, .T. ) ;
#7975=DIRECTION ( 'NONE',  ( 3.061276722312011504E-17, -1.000000000000000000, 0.000000000000000000 ) ) ;
#7977=CIRCLE ( 'NONE', #449, 7.500000000000007994 ) ;
#7980=ORIENTED_EDGE ( 'NONE', *, *, #3742, .F. ) ;
#7982=CARTESIAN_POINT ( 'NONE',  ( -381.3383124606481260, 66.03027902319438169, -136.7757352781387112 ) ) ;
#7985=VECTOR ( 'NONE', #5245, 1000.000000000000000 ) ;
#7986=CARTESIAN_POINT ( 'NONE',  ( -372.6862240691809234, 99.87440285508435522, -146.7032139785486038 ) ) ;
#7988=CARTESIAN_POINT ( 'NONE',  ( -371.5046744491019126, 60.13769991414361726, -107.9593700007184651 ) ) ;
#7991=EDGE_CURVE ( 'NONE', #4712, #7498, #2327, .T. ) ;
#7998=EDGE_LOOP ( 'NONE', ( #4217, #3504 ) ) ;
#8001=DIRECTION ( 'NONE',  ( -8.163404592832030268E-17, 1.000000000000000000, -0.000000000000000000 ) ) ;
#8005=AXIS2_PLACEMENT_3D ( 'NONE', #8596, #6556, #5627 ) ;
#8012=CARTESIAN_POINT ( 'NONE',  ( -374.7795003443170572, 87.57921835826481072, -95.35916363615964997 ) ) ;
#8014=VERTEX_POINT ( 'NONE', #11701 ) ;
#8015=DIRECTION ( 'NONE',  ( 3.061276722312011504E-17, -1.000000000000000000, 0.000000000000000000 ) ) ;
#8018=ORIENTED_EDGE ( 'NONE', *, *, #8880, .F. ) ;
#8019=CYLINDRICAL_SURFACE ( 'NONE', #10000, 7.500000000000007105 ) ;
#8029=MANIFOLD_SOLID_BREP ( 'Cut-Extrude4[1]', #2165 ) ;
#8032=CYLINDRICAL_SURFACE ( 'NONE', #10260, 5.000000000000004441 ) ;
#8045=CARTESIAN_POINT ( 'NONE',  ( -384.5742507613888392, 76.39205230857155016, -143.9146518029666311 ) ) ;
#8046=CARTESIAN_POINT ( 'NONE',  ( -371.7911309421997998, 102.9548155466288080, -142.7648159640167194 ) ) ;
#8058=DIRECTION ( 'NONE',  ( -1.000000000000000000, 0.000000000000000000, 0.000000000000000000 ) ) ;
#8061=CIRCLE ( 'NONE', #2734, 7.500000000000007994 ) ;
#8081=CARTESIAN_POINT ( 'NONE',  ( -262.5000000000000000, 139.9999999999999716, -126.4213562373076059 ) ) ;
#8096=CARTESIAN_POINT ( 'NONE',  ( -240.0000000000000000, 139.9999999999999716, -126.4213562373078190 ) ) ;
#8097=LINE ( 'NONE', #8154, #475 ) ;
#8099=ORIENTED_EDGE ( 'NONE', *, *, #9762, .F. ) ;
#8104=EDGE_CURVE ( 'NONE', #8014, #11084, #2510, .T. ) ;
#8112=ORIENTED_EDGE ( 'NONE', *, *, #5465, .T. ) ;
#8114=FACE_BOUND ( 'NONE', #2244, .T. ) ;
#8123=EDGE_LOOP ( 'NONE', ( #2905, #6801 ) ) ;
#8124=ADVANCED_FACE ( 'NONE', ( #6069 ), #9834, .F. ) ;
#8134=VERTEX_POINT ( 'NONE', #10948 ) ;
#8135=ADVANCED_FACE ( 'NONE', ( #5249 ), #7240, .F. ) ;
#8149=DIRECTION ( 'NONE',  ( 0.000000000000000000, 0.000000000000000000, 1.000000000000000000 ) ) ;
#8154=CARTESIAN_POINT ( 'NONE',  ( -202.4999999999999716, -9.213203435596478030, -126.4213562373080180 ) ) ;
#8158=ORIENTED_EDGE ( 'NONE', *, *, #903, .T. ) ;
#8160=DIRECTION ( 'NONE',  ( -8.163404592832030268E-17, 1.000000000000000000, -0.000000000000000000 ) ) ;
#8166=VERTEX_POINT ( 'NONE', #6129 ) ;
#8170=EDGE_LOOP ( 'NONE', ( #145, #3752, #4050, #11551 ) ) ;
#8175=CIRCLE ( 'NONE', #6399, 7.500000000000007105 ) ;
#8178=CARTESIAN_POINT ( 'NONE',  ( -369.9377146894910311, 55.86387605661327171, -127.6416088482251467 ) ) ;
#8181=CARTESIAN_POINT ( 'NONE',  ( 7.500000000000019540, 24.00000000000001421, -126.4213562373094959 ) ) ;
#8182=ORIENTED_EDGE ( 'NONE', *, *, #8722, .T. ) ;
#8184=VECTOR ( 'NONE', #4453, 1000.000000000000000 ) ;
#8201=DIRECTION ( 'NONE',  ( -8.163404592832031500E-17, 1.000000000000000000, 0.000000000000000000 ) ) ;
#8202=EDGE_CURVE ( 'NONE', #1855, #9681, #7264, .T. ) ;
#8209=CIRCLE ( 'NONE', #8604, 7.500000000000007105 ) ;
#8222=CARTESIAN_POINT ( 'NONE',  ( -270.0000000000000000, -9.213203435596478030, -126.4213562373076059 ) ) ;
#8224=CARTESIAN_POINT ( 'NONE',  ( -372.6850217215775274, 64.13912682578764191, -102.6824241675982989 ) ) ;
#8238=ORIENTED_EDGE ( 'NONE', *, *, #4594, .T. ) ;
#8249=CARTESIAN_POINT ( 'NONE',  ( -372.5380659305778295, 62.41370632951886677, -128.7741405147628200 ) ) ;
#8250=FACE_OUTER_BOUND ( 'NONE', #4660, .T. ) ;
#8251=VERTEX_POINT ( 'NONE', #9132 ) ;
#8254=COLOUR_RGB ( '', 0.09019608, 0.27058824, 0.51372549) ;
#8260=CARTESIAN_POINT ( 'NONE',  ( -828.8285638327206470, 78.67432280806529832, -144.4023295390027215 ) ) ;
#8262=CARTESIAN_POINT ( 'NONE',  ( -375.0216849847562344, 81.99049224892637255, -94.61449237475785878 ) ) ;
#8275=DIRECTION ( 'NONE',  ( 3.061276722312011504E-17, -1.000000000000000000, 0.000000000000000000 ) ) ;
#8278=EDGE_CURVE ( 'NONE', #6648, #10083, #2147, .T. ) ;
#8281=VERTEX_POINT ( 'NONE', #1420 ) ;
#8285=ORIENTED_EDGE ( 'NONE', *, *, #5684, .F. ) ;
#8305=ORIENTED_EDGE ( 'NONE', *, *, #1686, .F. ) ;
#8318=CARTESIAN_POINT ( 'NONE',  ( -379.2603478177108514, 62.16253007075349046, -127.3105118702911938 ) ) ;
#8321=CARTESIAN_POINT ( 'NONE',  ( -305.0000000000000568, 11.99999999999998224, -89.68077099980384048 ) ) ;
#8330=CARTESIAN_POINT ( 'NONE',  ( -825.1286147475018424, 83.51336106040476182, -144.6235354408670162 ) ) ;
#8335=DIRECTION ( 'NONE',  ( 0.000000000000000000, 1.000000000000000000, -0.000000000000000000 ) ) ;
#8337=AXIS2_PLACEMENT_3D ( 'NONE', #1767, #7328, #4615 ) ;
#8338=EDGE_CURVE ( 'NONE', #4125, #7035, #7164, .T. ) ;
#8339=CARTESIAN_POINT ( 'NONE',  ( -820.5035528205692117, 74.92619343081587147, -105.9719278460591596 ) ) ;
#8341=CARTESIAN_POINT ( 'NONE',  ( -821.7324155770269272, 74.13196894618555177, -143.0682369473086055 ) ) ;
#8344=CARTESIAN_POINT ( 'NONE',  ( -369.9928909712432983, 56.00132045696368976, -120.5003237462438221 ) ) ;
#8346=CARTESIAN_POINT ( 'NONE',  ( -381.0253547164383008, 98.60296799592514105, -113.5251504039077588 ) ) ;
#8347=ORIENTED_EDGE ( 'NONE', *, *, #4178, .T. ) ;
#8351=CYLINDRICAL_SURFACE ( 'NONE', #9381, 57.99999999999999289 ) ;
#8360=CARTESIAN_POINT ( 'NONE',  ( -372.4203662516890745, 101.9987822128686048, -123.8978246257192097 ) ) ;
#8364=DIRECTION ( 'NONE',  ( 1.000000000000000000, 0.000000000000000000, 0.000000000000000000 ) ) ;
#8368=CARTESIAN_POINT ( 'NONE',  ( -373.2167405728580434, 97.70338709260114740, -148.7255640766979354 ) ) ;
#8369=VERTEX_POINT ( 'NONE', #7102 ) ;
#8375=EDGE_CURVE ( 'NONE', #8983, #9395, #7347, .T. ) ;
#8380=VERTEX_POINT ( 'NONE', #9007 ) ;
#8382=CARTESIAN_POINT ( 'NONE',  ( -382.0430766089316421, 67.63206925129327374, -138.5972335451334629 ) ) ;
#8386=EDGE_CURVE ( 'NONE', #3022, #2997, #10004, .T. ) ;
#8391=CARTESIAN_POINT ( 'NONE',  ( -89.99999999999998579, 12.00000000000001421, -126.4213562373088564 ) ) ;
#8395=CIRCLE ( 'NONE', #10545, 7.500000000000007105 ) ;
#8396=CARTESIAN_POINT ( 'NONE',  ( -819.4849966174430165, 81.17290644373777297, -144.6655594550751402 ) ) ;
#8397=CIRCLE ( 'NONE', #9760, 7.500000000000007105 ) ;
#8400=CARTESIAN_POINT ( 'NONE',  ( -369.9107093661896215, 108.2030601565901549, -126.5620920014721094 ) ) ;
#8401=ORIENTED_EDGE ( 'NONE', *, *, #4594, .F. ) ;
#8403=CARTESIAN_POINT ( 'NONE',  ( -365.0000000000000568, 102.0000000000000142, -124.6807709998038405 ) ) ;
#8404=CARTESIAN_POINT ( 'NONE',  ( -379.7921418149276747, 53.60747417478052057, -114.9924028573224035 ) ) ;
#8408=CIRCLE ( 'NONE', #3863, 7.500000000000007994 ) ;
#8409=CARTESIAN_POINT ( 'NONE',  ( -819.4847856676369702, 76.17713329584734083, -105.5450962460538165 ) ) ;
#8411=CARTESIAN_POINT ( 'NONE',  ( -826.0729559276762757, 74.19411019796167750, -143.0951037527838139 ) ) ;
#8413=CARTESIAN_POINT ( 'NONE',  ( -373.0692867644656872, 65.64952826050301837, -148.1814920571080734 ) ) ;
#8415=CARTESIAN_POINT ( 'NONE',  ( -383.1555409210616290, 93.38962432455592477, -108.2374382966716837 ) ) ;
#8416=ORIENTED_EDGE ( 'NONE', *, *, #4786, .T. ) ;
#8420=FACE_OUTER_BOUND ( 'NONE', #10727, .T. ) ;
#8422=EDGE_LOOP ( 'NONE', ( #7811, #1770, #10400, #9545 ) ) ;
#8423=DIRECTION ( 'NONE',  ( -8.163404592832030268E-17, 1.000000000000000000, -0.000000000000000000 ) ) ;
#8424=CARTESIAN_POINT ( 'NONE',  ( -157.5000000000000000, -9.213203435596451385, -126.4213562373084301 ) ) ;
#8427=CARTESIAN_POINT ( 'NONE',  ( -305.0000000000000568, 24.00000000000000711, -159.6807709998038547 ) ) ;
#8438=EDGE_LOOP ( 'NONE', ( #10314, #2304, #2541, #11772 ) ) ;
#8445=CARTESIAN_POINT ( 'NONE',  ( -371.6769972486663960, 60.68164136501989248, -142.2120404103473561 ) ) ;
#8463=AXIS2_PLACEMENT_3D ( 'NONE', #1371, #7178, #7365 ) ;
#8464=CARTESIAN_POINT ( 'NONE',  ( -217.5000000000000000, -9.213203435596478030, -126.4213562373080180 ) ) ;
#8470=VECTOR ( 'NONE', #1478, 1000.000000000000000 ) ;
#8472=CARTESIAN_POINT ( 'NONE',  ( -37.50000000000000711, 152.0000000000000000, -126.4213562373092685 ) ) ;
#8473=CARTESIAN_POINT ( 'NONE',  ( -373.4274415647627166, 98.04483789281530903, -112.6589849898505236 ) ) ;
#8476=AXIS2_PLACEMENT_3D ( 'NONE', #174, #7724, #11850 ) ;
#8481=CIRCLE ( 'NONE', #3130, 35.00000000000000711 ) ;
#8490=ORIENTED_EDGE ( 'NONE', *, *, #4894, .F. ) ;
#8493=AXIS2_PLACEMENT_3D ( 'NONE', #7965, #1524, #2339 ) ;
#8494=ORIENTED_EDGE ( 'NONE', *, *, #3666, .F. ) ;
#8500=CARTESIAN_POINT ( 'NONE',  ( -374.4362727378983777, 73.12462464385868088, -152.9182541025093940 ) ) ;
#8502=CARTESIAN_POINT ( 'NONE',  ( -374.8916234221949821, 78.08292650439227600, -95.01254429865261386 ) ) ;
#8503=CYLINDRICAL_SURFACE ( 'NONE', #3907, 7.500000000000007105 ) ;
#8509=EDGE_CURVE ( 'NONE', #9164, #11519, #3916, .T. ) ;
#8511=CARTESIAN_POINT ( 'NONE',  ( -828.6712641482251911, 79.96111424986069949, -144.5792126457444908 ) ) ;
#8512=ADVANCED_FACE ( 'NONE', ( #8420 ), #4812, .F. ) ;
#8519=CARTESIAN_POINT ( 'NONE',  ( -150.0000000000000000, 24.00000000000001421, -126.4213562373084301 ) ) ;
#8522=CARTESIAN_POINT ( 'NONE',  ( -374.2864773846411595, 92.10316615029381637, -96.92210360129058699 ) ) ;
#8523=EDGE_CURVE ( 'NONE', #11140, #7745, #958, .T. ) ;
#8529=AXIS2_PLACEMENT_3D ( 'NONE', #2568, #528, #10113 ) ;
#8533=FACE_OUTER_BOUND ( 'NONE', #1212, .T. ) ;
#8538=DIRECTION ( 'NONE',  ( 1.000000000000000000, 0.000000000000000000, 0.000000000000000000 ) ) ;
#8541=CARTESIAN_POINT ( 'NONE',  ( -380.3309181785604665, 99.96675497247912290, -133.5619496204727454 ) ) ;
#8542=ORIENTED_EDGE ( 'NONE', *, *, #7842, .F. ) ;
#8548=DIRECTION ( 'NONE',  ( -2.040851148208007875E-17, 1.000000000000000000, 0.000000000000000000 ) ) ;
#8551=CARTESIAN_POINT ( 'NONE',  ( -384.8059386751791635, 78.06308572025466219, -144.3338303615605867 ) ) ;
#8553=CARTESIAN_POINT ( 'NONE',  ( -384.9624955846592229, 80.33371017125860192, -104.7475307242005869 ) ) ;
#8555=ORIENTED_EDGE ( 'NONE', *, *, #8104, .F. ) ;
#8560=DIRECTION ( 'NONE',  ( -1.000000000000000000, 0.000000000000000000, 0.000000000000000000 ) ) ;
#8563=CARTESIAN_POINT ( 'NONE',  ( -383.1733367470700955, 70.62324166987772855, -108.1910793484533997 ) ) ;
#8565=ORIENTED_EDGE ( 'NONE', *, *, #6388, .T. ) ;
#8568=LINE ( 'NONE', #6649, #5856 ) ;
#8570=EDGE_CURVE ( 'NONE', #6627, #957, #42, .T. ) ;
#8571=DIRECTION ( 'NONE',  ( -8.163404592832030268E-17, 1.000000000000000000, -0.000000000000000000 ) ) ;
#8572=CYLINDRICAL_SURFACE ( 'NONE', #9565, 7.500000000000007105 ) ;
#8575=FACE_BOUND ( 'NONE', #11654, .T. ) ;
#8589=CARTESIAN_POINT ( 'NONE',  ( -157.5000000000000000, -9.213203435596451385, -126.4213562373084301 ) ) ;
#8590=CARTESIAN_POINT ( 'NONE',  ( -82.49999999999997158, 24.00000000000001421, -126.4213562373088564 ) ) ;
#8596=CARTESIAN_POINT ( 'NONE',  ( -90.00000000000000000, 139.9999999999999716, -126.4213562373088564 ) ) ;
#8599=CARTESIAN_POINT ( 'NONE',  ( -372.7918232332913817, 100.6587063813212524, -131.9323245634151647 ) ) ;
#8603=ADVANCED_FACE ( 'NONE', ( #4184 ), #400, .F. ) ;
#8604=AXIS2_PLACEMENT_3D ( 'NONE', #6222, #10106, #3358 ) ;
#8605=EDGE_LOOP ( 'NONE', ( #4794, #1138, #11320, #9190 ) ) ;
#8606=B_SPLINE_CURVE_WITH_KNOTS ( 'NONE', 3,
 ( #4568, #11976, #3494, #6345, #10119, #8344, #7408, #3552, #726, #1652, #5412, #11182, #9191, #4504, #7342, #11113, #6478, #10252, #4635, #1786, #5548, #865, #8413, #12176, #3692, #7469, #2774, #6538, #10306, #8760, #7768, #10549, #35, #153, #6659, #5914, #9566, #4921 ),
 .UNSPECIFIED., .F., .F.,
 ( 4, 2, 2, 2, 2, 2, 2, 2, 2, 2, 2, 2, 2, 2, 2, 2, 2, 2, 4 ),
 ( 0.07998895219617635499, 0.08341829896746193185, 0.08513297235310469946, 0.08684764573874746707, 0.09370633928131860690, 0.09713568605260422539, 0.1005650328238898439, 0.1039943795951754624, 0.1057090529808182716, 0.1074237263664610809, 0.1142824199090320403, 0.1177117666803174645, 0.1211411134516029164, 0.1228557868372455869, 0.1245704602228882713, 0.1279998069941736261, 0.1314291537654590225, 0.1331438271511017069, 0.1348585005367443912 ),
 .UNSPECIFIED. ) ;
#8608=FACE_BOUND ( 'NONE', #5090, .T. ) ;
#8610=ORIENTED_EDGE ( 'NONE', *, *, #9494, .T. ) ;
#8611=CARTESIAN_POINT ( 'NONE',  ( -374.7039800877403763, 74.36633201333150112, -143.2283958171015854 ) ) ;
#8613=CARTESIAN_POINT ( 'NONE',  ( -374.9671836365860713, 79.81299459977714150, -94.78091058644133682 ) ) ;
#8614=DIRECTION ( 'NONE',  ( 1.000000000000000000, 0.000000000000000000, 0.000000000000000000 ) ) ;
#8627=CARTESIAN_POINT ( 'NONE',  ( -384.8558507370726147, 78.74686981056612467, -104.9381817955416096 ) ) ;
#8634=DIRECTION ( 'NONE',  ( 3.061276722312011504E-17, -1.000000000000000000, 0.000000000000000000 ) ) ;
#8643=CARTESIAN_POINT ( 'NONE',  ( -374.7080949166565347, 88.40015326679682062, -95.58188032217027796 ) ) ;
#8649=DIRECTION ( 'NONE',  ( -8.163404592832030268E-17, 1.000000000000000000, -0.000000000000000000 ) ) ;
#8655=CARTESIAN_POINT ( 'NONE',  ( -375.0000000000000000, 83.13026420090928070, -94.68077099980384048 ) ) ;
#8661=EDGE_LOOP ( 'NONE', ( #4774, #11137 ) ) ;
#8672=DIRECTION ( 'NONE',  ( 0.000000000000000000, 1.000000000000000000, 0.000000000000000000 ) ) ;
#8674=CARTESIAN_POINT ( 'NONE',  ( 1.959217102279688941E-15, 139.9999999999999716, -126.4213562373094959 ) ) ;
#8676=ORIENTED_EDGE ( 'NONE', *, *, #10025, .T. ) ;
#8677=CARTESIAN_POINT ( 'NONE',  ( -383.2504773128821398, 70.84834670873947005, -141.3339299216349616 ) ) ;
#8679=CARTESIAN_POINT ( 'NONE',  ( -372.9799184754957082, 65.30137661730785226, -101.5283204515378088 ) ) ;
#8684=CARTESIAN_POINT ( 'NONE',  ( -375.0000000000000000, 81.99999999999995737, -89.68077099980384048 ) ) ;
#8691=CARTESIAN_POINT ( 'NONE',  ( -384.4864278086921558, 75.86462062201600531, -105.6083542711734680 ) ) ;
#8699=FACE_BOUND ( 'NONE', #8737, .T. ) ;
#8701=ORIENTED_EDGE ( 'NONE', *, *, #6780, .T. ) ;
#8707=EDGE_CURVE ( 'NONE', #7292, #3585, #11675, .T. ) ;
#8710=CYLINDRICAL_SURFACE ( 'NONE', #7776, 7.500000000000007105 ) ;
#8711=CARTESIAN_POINT ( 'NONE',  ( -819.8468830326148691, 81.71630402067583532, -104.6809196082601119 ) ) ;
#8720=AXIS2_PLACEMENT_3D ( 'NONE', #2104, #2963, #6725 ) ;
#8722=EDGE_CURVE ( 'NONE', #3971, #2594, #9046, .T. ) ;
#8728=CARTESIAN_POINT ( 'NONE',  ( -202.4999999999999716, -9.213203435596478030, -126.4213562373080180 ) ) ;
#8730=CARTESIAN_POINT ( 'NONE',  ( -374.9896482698936779, 80.71982717203331958, -154.6492122816839299 ) ) ;
#8731=DIRECTION ( 'NONE',  ( 1.000000000000000000, 0.000000000000000000, 0.000000000000000000 ) ) ;
#8732=CARTESIAN_POINT ( 'NONE',  ( -374.9143915958317166, 78.51216652322804634, -94.94260781757940038 ) ) ;
#8735=VERTEX_POINT ( 'NONE', #3076 ) ;
#8736=AXIS2_PLACEMENT_3D ( 'NONE', #3377, #479, #6241 ) ;
#8737=EDGE_LOOP ( 'NONE', ( #8347, #4742 ) ) ;
#8744=CARTESIAN_POINT ( 'NONE',  ( -379.8999661783463466, 63.26100480178833863, -117.6669381337575544 ) ) ;
#8745=ORIENTED_EDGE ( 'NONE', *, *, #4565, .T. ) ;
#8746=DIRECTION ( 'NONE',  ( 0.000000000000000000, 0.000000000000000000, 1.000000000000000000 ) ) ;
#8751=ORIENTED_EDGE ( 'NONE', *, *, #2319, .F. ) ;
#8759=EDGE_LOOP ( 'NONE', ( #1744, #1607, #2434, #11665, #2265, #2961, #4595, #8542, #2114, #758 ) ) ;
#8760=CARTESIAN_POINT ( 'NONE',  ( -374.4501075384643514, 73.18187568907286789, -152.9657676401715491 ) ) ;
#8764=ORIENTED_EDGE ( 'NONE', *, *, #2772, .T. ) ;
#8768=ORIENTED_EDGE ( 'NONE', *, *, #105, .T. ) ;
#8770=CARTESIAN_POINT ( 'NONE',  ( -821.6103028745218353, 83.16718542005921222, -104.7144644823254822 ) ) ;
#8774=ORIENTED_EDGE ( 'NONE', *, *, #6014, .T. ) ;
#8778=AXIS2_PLACEMENT_3D ( 'NONE', #3737, #10475, #11464 ) ;
#8790=DIRECTION ( 'NONE',  ( 3.061276722312011504E-17, -1.000000000000000000, 0.000000000000000000 ) ) ;
#8791=CARTESIAN_POINT ( 'NONE',  ( -381.0053422273798560, 65.34300945855264331, -113.5331703338095082 ) ) ;
#8795=VECTOR ( 'NONE', #589, 1000.000000000000000 ) ;
#8801=CARTESIAN_POINT ( 'NONE',  ( -372.7937968025734108, 63.34872752676778873, -117.4098597798181629 ) ) ;
#8802=CYLINDRICAL_SURFACE ( 'NONE', #5584, 7.500000000000007105 ) ;
#8810=FACE_OUTER_BOUND ( 'NONE', #1497, .T. ) ;
#8814=DIRECTION ( 'NONE',  ( -1.000000000000000000, 0.000000000000000000, 0.000000000000000000 ) ) ;
#8821=ADVANCED_FACE ( 'NONE', ( #10762 ), #1492, .T. ) ;
#8827=CARTESIAN_POINT ( 'NONE',  ( -818.8614429351425770, 78.01598473359217678, -144.2826642275888105 ) ) ;
#8829=DIRECTION ( 'NONE',  ( -8.163404592832031500E-17, 1.000000000000000000, 0.000000000000000000 ) ) ;
#8831=FACE_BOUND ( 'NONE', #2789, .T. ) ;
#8836=AXIS2_PLACEMENT_3D ( 'NONE', #7624, #7560, #4783 ) ;
#8839=DIRECTION ( 'NONE',  ( -8.163404592832030268E-17, 1.000000000000000000, -0.000000000000000000 ) ) ;
#8844=VECTOR ( 'NONE', #2902, 1000.000000000000000 ) ;
#8845=CARTESIAN_POINT ( 'NONE',  ( 1.414009460465297036E-14, -9.213203435596451385, -126.4213562373094959 ) ) ;
#8846=CARTESIAN_POINT ( 'NONE',  ( -210.0000000000000000, 24.00000000000000711, -126.4213562373080180 ) ) ;
#8857=CARTESIAN_POINT ( 'NONE',  ( -370.0761506609951539, 56.20937627747883880, -118.7459503409855301 ) ) ;
#8859=CARTESIAN_POINT ( 'NONE',  ( -382.0049300299783681, 96.47769172040968044, -110.8343367138896838 ) ) ;
#8860=CARTESIAN_POINT ( 'NONE',  ( -22.49999999999997868, 12.00000000000001776, -126.4213562373092685 ) ) ;
#8861=VERTEX_POINT ( 'NONE', #10820 ) ;
#8862=ORIENTED_EDGE ( 'NONE', *, *, #11586, .F. ) ;
#8869=DIRECTION ( 'NONE',  ( -8.163404592832030268E-17, 1.000000000000000000, -0.000000000000000000 ) ) ;
#8878=CARTESIAN_POINT ( 'NONE',  ( -120.0000000000000000, 152.0000000000000000, -126.4213562373086575 ) ) ;
#8880=EDGE_CURVE ( 'NONE', #7697, #11231, #5189, .T. ) ;
#8882=CARTESIAN_POINT ( 'NONE',  ( -828.3277261219641332, 80.87986238895008739, -104.7098637035477964 ) ) ;
#8883=DIRECTION ( 'NONE',  ( 0.000000000000000000, 0.000000000000000000, 1.000000000000000000 ) ) ;
#8884=DIRECTION ( 'NONE',  ( 1.000000000000000000, -0.000000000000000000, -0.000000000000000000 ) ) ;
#8893=CARTESIAN_POINT ( 'NONE',  ( -384.7383783008219211, 77.53302683473108914, -144.2117537804176095 ) ) ;
#8894=CARTESIAN_POINT ( 'NONE',  ( -373.4439786919718927, 96.68931900664449586, -149.5563464679744072 ) ) ;
#8906=DIRECTION ( 'NONE',  ( 0.000000000000000000, 0.000000000000000000, 1.000000000000000000 ) ) ;
#8909=CIRCLE ( 'NONE', #12090, 7.500000000000007105 ) ;
#8918=VERTEX_POINT ( 'NONE', #2534 ) ;
#8920=ADVANCED_FACE ( 'NONE', ( #3515 ), #4592, .F. ) ;
#8921=SHAPE_REPRESENTATION_RELATIONSHIP ( 'NONE' , 'NONE' ,  #6140, #2640 ) ;
#8922=EDGE_LOOP ( 'NONE', ( #3091, #1684 ) ) ;
#8923=CARTESIAN_POINT ( 'NONE',  ( 0.000000000000000000, 24.00000000000001776, -89.68077099980384048 ) ) ;
#8932=LINE ( 'NONE', #11676, #7294 ) ;
#8937=DIRECTION ( 'NONE',  ( 3.061276722312011504E-17, -1.000000000000000000, 0.000000000000000000 ) ) ;
#8939=DIRECTION ( 'NONE',  ( 1.000000000000000000, 0.000000000000000000, 0.000000000000000000 ) ) ;
#8944=EDGE_CURVE ( 'NONE', #11420, #7745, #820, .T. ) ;
#8953=CARTESIAN_POINT ( 'NONE',  ( 0.000000000000000000, 12.00000000000001776, -159.6807709998038547 ) ) ;
#8956=ORIENTED_EDGE ( 'NONE', *, *, #401, .T. ) ;
#8958=CARTESIAN_POINT ( 'NONE',  ( -375.0000000000000568, 81.99999999999994316, -154.6807709998039115 ) ) ;
#8960=CIRCLE ( 'NONE', #6608, 7.500000000000007105 ) ;
#8961=DIRECTION ( 'NONE',  ( 0.000000000000000000, 0.000000000000000000, 1.000000000000000000 ) ) ;
#8966=ORIENTED_EDGE ( 'NONE', *, *, #5400, .F. ) ;
#8973=ORIENTED_EDGE ( 'NONE', *, *, #7693, .T. ) ;
#8975=CARTESIAN_POINT ( 'NONE',  ( -380.4056020936891969, 99.82458448124143047, -115.5361751508218759 ) ) ;
#8977=CIRCLE ( 'NONE', #9972, 69.99999999999998579 ) ;
#8979=CARTESIAN_POINT ( 'NONE',  ( -305.0000000000000568, 139.9999999999999716, -159.6807709998038547 ) ) ;
#8980=CARTESIAN_POINT ( 'NONE',  ( -217.5000000000000000, 151.9999999999999716, -126.4213562373080180 ) ) ;
#8982=DIRECTION ( 'NONE',  ( -1.000000000000000000, -3.061276722312011504E-17, -0.000000000000000000 ) ) ;
#8983=VERTEX_POINT ( 'NONE', #2728 ) ;
#8986=ORIENTED_EDGE ( 'NONE', *, *, #10817, .F. ) ;
#8987=DIRECTION ( 'NONE',  ( -1.000000000000000000, 0.000000000000000000, 0.000000000000000000 ) ) ;
#8997=DIRECTION ( 'NONE',  ( 0.000000000000000000, 1.000000000000000000, 0.000000000000000000 ) ) ;
#9000=CARTESIAN_POINT ( 'NONE',  ( -270.0000000000000000, 139.9999999999999716, -126.4213562373076059 ) ) ;
#9003=ORIENTED_EDGE ( 'NONE', *, *, #9358, .T. ) ;
#9004=DIRECTION ( 'NONE',  ( 2.040851148208007875E-17, -1.000000000000000000, -0.000000000000000000 ) ) ;
#9007=CARTESIAN_POINT ( 'NONE',  ( -127.5000000000000000, 139.9999999999999716, -126.4213562373086575 ) ) ;
#9015=CARTESIAN_POINT ( 'NONE',  ( -379.7887390581964837, 100.9343252097582422, -131.1221473163307678 ) ) ;
#9016=EDGE_CURVE ( 'NONE', #4282, #7284, #1608, .T. ) ;
#9017=CARTESIAN_POINT ( 'NONE',  ( -374.9550661767995621, 84.88126776701597009, -154.5446018065266287 ) ) ;
#9022=DIRECTION ( 'NONE',  ( -8.163404592832030268E-17, 1.000000000000000000, -0.000000000000000000 ) ) ;
#9033=CARTESIAN_POINT ( 'NONE',  ( -172.5000000000000000, 151.9999999999999716, -126.4213562373082453 ) ) ;
#9035=ORIENTED_EDGE ( 'NONE', *, *, #7129, .T. ) ;
#9044=CARTESIAN_POINT ( 'NONE',  ( -37.50000000000000711, 139.9999999999999716, -126.4213562373092685 ) ) ;
#9045=CARTESIAN_POINT ( 'NONE',  ( -374.8589991914415123, 86.47510645258195439, -95.11294974172253092 ) ) ;
#9046=CIRCLE ( 'NONE', #10436, 7.500000000000007105 ) ;
#9047=CARTESIAN_POINT ( 'NONE',  ( 7.500000000000022204, -9.213203435596451385, -126.4213562373094959 ) ) ;
#9048=CARTESIAN_POINT ( 'NONE',  ( 0.000000000000000000, 0.000000000000000000, 0.000000000000000000 ) ) ;
#9049=ORIENTED_EDGE ( 'NONE', *, *, #11755, .T. ) ;
#9053=ORIENTED_EDGE ( 'NONE', *, *, #6462, .F. ) ;
#9061=DIRECTION ( 'NONE',  ( 1.000000000000000000, 0.000000000000000000, 0.000000000000000000 ) ) ;
#9071=DIRECTION ( 'NONE',  ( 0.000000000000000000, 0.000000000000000000, 1.000000000000000000 ) ) ;
#9074=VERTEX_POINT ( 'NONE', #9214 ) ;
#9081=DIRECTION ( 'NONE',  ( 2.040851148208007875E-17, -1.000000000000000000, -0.000000000000000000 ) ) ;
#9088=ORIENTED_EDGE ( 'NONE', *, *, #391, .F. ) ;
#9089=ORIENTED_EDGE ( 'NONE', *, *, #11969, .F. ) ;
#9093=CARTESIAN_POINT ( 'NONE',  ( -372.5604626478378805, 62.49331231609644988, -129.1428628536290262 ) ) ;
#9094=CYLINDRICAL_SURFACE ( 'NONE', #4984, 7.500000000000007105 ) ;
#9102=DIRECTION ( 'NONE',  ( -8.163404592832031500E-17, 1.000000000000000000, 0.000000000000000000 ) ) ;
#9107=ADVANCED_FACE ( 'NONE', ( #537 ), #4319, .F. ) ;
#9112=LINE ( 'NONE', #6277, #8795 ) ;
#9124=CARTESIAN_POINT ( 'NONE',  ( -824.4866663711917454, 83.64159454339579725, -104.7481522953014235 ) ) ;
#9127=VERTEX_POINT ( 'NONE', #11858 ) ;
#9130=CYLINDRICAL_SURFACE ( 'NONE', #5964, 7.500000000000007105 ) ;
#9132=CARTESIAN_POINT ( 'NONE',  ( -305.0000000000000568, 151.9999999999999716, -89.68077099980384048 ) ) ;
#9137=ORIENTED_EDGE ( 'NONE', *, *, #3666, .T. ) ;
#9139=CARTESIAN_POINT ( 'NONE',  ( -379.1619848709565872, 61.99999999999991473, -125.8727444633825883 ) ) ;
#9146=ORIENTED_EDGE ( 'NONE', *, *, #6406, .F. ) ;
#9159=ORIENTED_EDGE ( 'NONE', *, *, #11803, .F. ) ;
#9160=CARTESIAN_POINT ( 'NONE',  ( -370.6591228199823718, 57.71959721323136705, -136.2503380851910890 ) ) ;
#9161=FACE_OUTER_BOUND ( 'NONE', #5004, .T. ) ;
#9164=VERTEX_POINT ( 'NONE', #4197 ) ;
#9166=EDGE_CURVE ( 'NONE', #9681, #1855, #6865, .T. ) ;
#9167=AXIS2_PLACEMENT_3D ( 'NONE', #2168, #4423, #9867 ) ;
#9174=DIRECTION ( 'NONE',  ( -1.000000000000000000, 0.000000000000000000, 0.000000000000000000 ) ) ;
#9176=CIRCLE ( 'NONE', #288, 7.500000000000007105 ) ;
#9187=CIRCLE ( 'NONE', #700, 7.500000000000020428 ) ;
#9190=ORIENTED_EDGE ( 'NONE', *, *, #9494, .F. ) ;
#9191=CARTESIAN_POINT ( 'NONE',  ( -370.3936982783733924, 57.02401252216581184, -133.9834721354013993 ) ) ;
#9197=DIRECTION ( 'NONE',  ( -8.163404592832030268E-17, 1.000000000000000000, -0.000000000000000000 ) ) ;
#9199=CARTESIAN_POINT ( 'NONE',  ( -305.0000000000000568, 81.99999999999995737, -89.68077099980384048 ) ) ;
#9201=ORIENTED_EDGE ( 'NONE', *, *, #1229, .T. ) ;
#9214=CARTESIAN_POINT ( 'NONE',  ( -97.49999999999998579, 12.00000000000001421, -126.4213562373088564 ) ) ;
#9218=CIRCLE ( 'NONE', #3098, 7.500000000000007105 ) ;
#9219=VERTEX_POINT ( 'NONE', #4267 ) ;
#9222=LINE ( 'NONE', #2671, #10343 ) ;
#9226=CARTESIAN_POINT ( 'NONE',  ( -371.9994406452410090, 61.71775825474107791, -143.7502050151522894 ) ) ;
#9230=CARTESIAN_POINT ( 'NONE',  ( -52.49999999999999289, 152.0000000000000000, -126.4213562373090696 ) ) ;
#9231=AXIS2_PLACEMENT_3D ( 'NONE', #2476, #9022, #1550 ) ;
#9239=EDGE_LOOP ( 'NONE', ( #9853, #1090 ) ) ;
#9240=AXIS2_PLACEMENT_3D ( 'NONE', #8096, #735, #9071 ) ;
#9243=CARTESIAN_POINT ( 'NONE',  ( -7.500000000000007105, 139.9999999999999716, -126.4213562373094959 ) ) ;
#9244=VERTEX_POINT ( 'NONE', #11801 ) ;
#9251=CARTESIAN_POINT ( 'NONE',  ( -824.1700714248495387, 73.67466183167371696, -106.4959216872580186 ) ) ;
#9254=ORIENTED_EDGE ( 'NONE', *, *, #11969, .T. ) ;
#9255=EDGE_LOOP ( 'NONE', ( #11975, #2987, #8158, #2005 ) ) ;
#9257=CARTESIAN_POINT ( 'NONE',  ( -373.5671007695220283, 97.39601910195885637, -111.8308065815015766 ) ) ;
#9267=EDGE_CURVE ( 'NONE', #9219, #10646, #4878, .T. ) ;
#9270=ADVANCED_FACE ( 'NONE', ( #5233 ), #6053, .T. ) ;
#9275=CARTESIAN_POINT ( 'NONE',  ( -369.8922502829638574, 108.2488063532000098, -123.6482589490543376 ) ) ;
#9279=LINE ( 'NONE', #817, #2668 ) ;
#9281=CARTESIAN_POINT ( 'NONE',  ( -52.49999999999997868, 12.00000000000001421, -126.4213562373090696 ) ) ;
#9283=CARTESIAN_POINT ( 'NONE',  ( -372.4866396559332316, 100.6260255300948501, -145.9099802644697661 ) ) ;
#9287=ORIENTED_EDGE ( 'NONE', *, *, #8509, .T. ) ;
#9293=CARTESIAN_POINT ( 'NONE',  ( -381.2022825699808664, 65.75744103998614776, -136.3682839401687943 ) ) ;
#9297=ORIENTED_EDGE ( 'NONE', *, *, #10821, .T. ) ;
#9302=CARTESIAN_POINT ( 'NONE',  ( -270.0000000000000000, 12.00000000000001066, -126.4213562373076059 ) ) ;
#9306=CARTESIAN_POINT ( 'NONE',  ( -826.0529305544605450, 83.16438776978687031, -144.6472496521799371 ) ) ;
#9308=CARTESIAN_POINT ( 'NONE',  ( -370.4017534246571586, 106.9526614274764853, -115.3486010405474929 ) ) ;
#9313=DIRECTION ( 'NONE',  ( -1.000000000000000000, 0.000000000000000000, 0.000000000000000000 ) ) ;
#9318=CARTESIAN_POINT ( 'NONE',  ( -828.5731535248124828, 77.06390383656750487, -144.0645491675084884 ) ) ;
#9321=EDGE_LOOP ( 'NONE', ( #11834, #322 ) ) ;
#9324=CARTESIAN_POINT ( 'NONE',  ( -383.9019967062238834, 90.88042285000165066, -106.7131948037297349 ) ) ;
#9326=ORIENTED_EDGE ( 'NONE', *, *, #8523, .T. ) ;
#9334=LINE ( 'NONE', #10130, #1432 ) ;
#9341=ORIENTED_EDGE ( 'NONE', *, *, #4405, .F. ) ;
#9348=PRODUCT_DEFINITION ( 'UNKNOWN', '', #6834, #2087 ) ;
#9353=AXIS2_PLACEMENT_3D ( 'NONE', #7460, #3610, #9313 ) ;
#9355=CARTESIAN_POINT ( 'NONE',  ( -372.7850951469527558, 63.30985991596471507, -132.0026127303325438 ) ) ;
#9358=EDGE_CURVE ( 'NONE', #8251, #9588, #12181, .T. ) ;
#9360=AXIS2_PLACEMENT_3D ( 'NONE', #981, #4302, #7076 ) ;
#9361=AXIS2_PLACEMENT_3D ( 'NONE', #3385, #555, #9894 ) ;
#9366=CARTESIAN_POINT ( 'NONE',  ( -29.99999999999998579, -9.213203435596451385, -126.4213562373092685 ) ) ;
#9371=CARTESIAN_POINT ( 'NONE',  ( -818.8285638327206470, 78.67432280806529832, -144.4023295390026931 ) ) ;
#9374=CARTESIAN_POINT ( 'NONE',  ( -371.1191838156116773, 105.0141530621877166, -110.0650553684051403 ) ) ;
#9377=LINE ( 'NONE', #11475, #1356 ) ;
#9381=AXIS2_PLACEMENT_3D ( 'NONE', #9199, #2890, #12115 ) ;
#9387=CARTESIAN_POINT ( 'NONE',  ( -374.7973491424790495, 88.50727265276420042, -105.6931112893597771 ) ) ;
#9394=VERTEX_POINT ( 'NONE', #6348 ) ;
#9395=VERTEX_POINT ( 'NONE', #3622 ) ;
#9398=CARTESIAN_POINT ( 'NONE',  ( -37.50000000000000000, 24.00000000000001421, -126.4213562373092685 ) ) ;
#9405=CARTESIAN_POINT ( 'NONE',  ( -373.4654644648271073, 97.87726989067260774, -136.9400350704844129 ) ) ;
#9414=DIRECTION ( 'NONE',  ( 2.040851148208007875E-17, -1.000000000000000000, -0.000000000000000000 ) ) ;
#9417=CARTESIAN_POINT ( 'NONE',  ( -384.1670479773604256, 74.31760017581927968, -143.1493696165661333 ) ) ;
#9419=CARTESIAN_POINT ( 'NONE',  ( -372.8161565995750948, 64.64827838876098554, -102.1643297174437635 ) ) ;
#9424=AXIS2_PLACEMENT_3D ( 'NONE', #7134, #6148, #582 ) ;
#9430=B_SPLINE_CURVE_WITH_KNOTS ( 'NONE', 3,
 ( #8958, #4153, #9017, #7868, #11697, #11641, #3159, #488, #10699, #3210, #10759, #9830, #2409, #8894, #419, #4209, #7986, #11759, #7045, #4277, #8046, #11815, #3331, #7110, #10874, #5244 ),
 .UNSPECIFIED., .F., .F.,
 ( 4, 2, 2, 2, 2, 2, 2, 2, 2, 2, 2, 2, 4 ),
 ( 0.1348585005367443912, 0.1392389232406545940, 0.1414291345926096954, 0.1425242402685872323, 0.1436193459445647691, 0.1479997686484748332, 0.1501899800004299068, 0.1523801913523849527, 0.1567606140562951278, 0.1589508254082501737, 0.1611410367602052196, 0.1655214594641153114, 0.1699018821680253755 ),
 .UNSPECIFIED. ) ;
#9432=CARTESIAN_POINT ( 'NONE',  ( -828.7978644797661900, 79.31746325908696349, -144.5027040960656564 ) ) ;
#9439=CARTESIAN_POINT ( 'NONE',  ( -217.5000000000000000, -9.213203435596478030, -126.4213562373080180 ) ) ;
#9442=CYLINDRICAL_SURFACE ( 'NONE', #4822, 7.500000000000007105 ) ;
#9444=ORIENTED_EDGE ( 'NONE', *, *, #401, .F. ) ;
#9445=CYLINDRICAL_SURFACE ( 'NONE', #9360, 7.500000000000007105 ) ;
#9446=CARTESIAN_POINT ( 'NONE',  ( -373.6858788323772842, 95.50525450785576709, -98.95117123207425891 ) ) ;
#9448=VECTOR ( 'NONE', #8571, 1000.000000000000000 ) ;
#9449=DIRECTION ( 'NONE',  ( -1.000000000000000000, 0.000000000000000000, 0.000000000000000000 ) ) ;
#9452=VERTEX_POINT ( 'NONE', #7379 ) ;
#9453=DIRECTION ( 'NONE',  ( -1.000000000000000000, 0.000000000000000000, 0.000000000000000000 ) ) ;
#9465=ORIENTED_EDGE ( 'NONE', *, *, #6820, .F. ) ;
#9470=DIRECTION ( 'NONE',  ( -8.163404592832030268E-17, 1.000000000000000000, -0.000000000000000000 ) ) ;
#9473=ADVANCED_FACE ( 'NONE', ( #5450 ), #11085, .F. ) ;
#9474=CARTESIAN_POINT ( 'NONE',  ( -374.9351506289129361, 85.78662242748217182, -144.3442421662540198 ) ) ;
#9476=CARTESIAN_POINT ( 'NONE',  ( -374.2976682315979247, 70.77949302303818513, -108.0449445377915225 ) ) ;
#9481=DIRECTION ( 'NONE',  ( -8.163404592832030268E-17, 1.000000000000000000, -0.000000000000000000 ) ) ;
#9482=CARTESIAN_POINT ( 'NONE',  ( -67.49999999999998579, -9.213203435596451385, -126.4213562373090696 ) ) ;
#9487=ORIENTED_EDGE ( 'NONE', *, *, #4178, .F. ) ;
#9488=CARTESIAN_POINT ( 'NONE',  ( -820.5266942580627756, 82.43260598963586006, -144.6763645173219004 ) ) ;
#9494=EDGE_CURVE ( 'NONE', #9074, #966, #7629, .T. ) ;
#9496=DIRECTION ( 'NONE',  ( -1.000000000000000000, 0.000000000000000000, 0.000000000000000000 ) ) ;
#9500=DIRECTION ( 'NONE',  ( 0.000000000000000000, 1.000000000000000000, -0.000000000000000000 ) ) ;
#9504=CARTESIAN_POINT ( 'NONE',  ( -374.5716219028437308, 90.99737113659554666, -106.7529307625888606 ) ) ;
#9521=CARTESIAN_POINT ( 'NONE',  ( -373.2951768170237301, 97.35898663981262757, -149.0144453010688039 ) ) ;
#9525=EDGE_LOOP ( 'NONE', ( #2160, #1849, #10536, #2897 ) ) ;
#9527=CARTESIAN_POINT ( 'NONE',  ( -120.0000000000000000, 139.9999999999999716, -126.4213562373086575 ) ) ;
#9532=CARTESIAN_POINT ( 'NONE',  ( -373.4691676486093570, 67.36345505517621746, -149.6605093826277084 ) ) ;
#9533=DIRECTION ( 'NONE',  ( -8.163404592832031500E-17, 1.000000000000000000, 0.000000000000000000 ) ) ;
#9534=CARTESIAN_POINT ( 'NONE',  ( -382.5041789709763407, 68.77964067713233476, -109.6698101448797615 ) ) ;
#9537=ORIENTED_EDGE ( 'NONE', *, *, #4514, .F. ) ;
#9538=ADVANCED_FACE ( 'NONE', ( #10526 ), #10589, .F. ) ;
#9539=EDGE_LOOP ( 'NONE', ( #2575, #518 ) ) ;
#9545=ORIENTED_EDGE ( 'NONE', *, *, #10982, .F. ) ;
#9553=DIRECTION ( 'NONE',  ( 2.040851148208007875E-17, -1.000000000000000000, -0.000000000000000000 ) ) ;
#9558=FACE_BOUND ( 'NONE', #1157, .T. ) ;
#9565=AXIS2_PLACEMENT_3D ( 'NONE', #4117, #5841, #5777 ) ;
#9566=CARTESIAN_POINT ( 'NONE',  ( -375.0000000000000000, 81.43281243045049678, -154.6807709998038263 ) ) ;
#9574=FACE_OUTER_BOUND ( 'NONE', #5130, .T. ) ;
#9576=CARTESIAN_POINT ( 'NONE',  ( -374.5762240358420740, 89.76870905692126712, -95.99562579782801208 ) ) ;
#9580=CARTESIAN_POINT ( 'NONE',  ( -370.0786918602308333, 107.7875646358821200, -118.7374980023263049 ) ) ;
#9588=VERTEX_POINT ( 'NONE', #8684 ) ;
#9594=CARTESIAN_POINT ( 'NONE',  ( -374.8301963407180892, 76.83280000780887065, -154.1603600426035428 ) ) ;
#9596=CARTESIAN_POINT ( 'NONE',  ( -374.0135547283281312, 68.94350272267550395, -109.4340150406342218 ) ) ;
#9608=CIRCLE ( 'NONE', #4284, 7.500000000000020428 ) ;
#9614=LINE ( 'NONE', #8464, #5690 ) ;
#9622=ORIENTED_EDGE ( 'NONE', *, *, #10982, .T. ) ;
#9624=EDGE_CURVE ( 'NONE', #11206, #4244, #6643, .T. ) ;
#9633=CARTESIAN_POINT ( 'NONE',  ( -217.5000000000000000, 139.9999999999999716, -126.4213562373080180 ) ) ;
#9635=CARTESIAN_POINT ( 'NONE',  ( -380.2012603716702870, 100.1962551005152733, -116.3549404919051113 ) ) ;
#9638=DIRECTION ( 'NONE',  ( -8.163404592832030268E-17, 1.000000000000000000, -0.000000000000000000 ) ) ;
#9640=EDGE_LOOP ( 'NONE', ( #8966, #4295 ) ) ;
#9646=CARTESIAN_POINT ( 'NONE',  ( -180.0000000000000000, 139.9999999999999716, -126.4213562373082453 ) ) ;
#9648=VECTOR ( 'NONE', #10741, 1000.000000000000000 ) ;
#9651=AXIS2_PLACEMENT_3D ( 'NONE', #10077, #11999, #11134 ) ;
#9654=CARTESIAN_POINT ( 'NONE',  ( -379.7887390581964837, 100.9343252097582564, -131.1221473163307678 ) ) ;
#9656=LINE ( 'NONE', #8728, #5832 ) ;
#9657=CARTESIAN_POINT ( 'NONE',  ( -384.9995590721709959, 82.68011010844932684, -144.6800286746663460 ) ) ;
#9659=CARTESIAN_POINT ( 'NONE',  ( -384.4111993152493483, 75.51142861137186912, -105.7511216177616120 ) ) ;
#9667=AXIS2_PLACEMENT_3D ( 'NONE', #6409, #1584, #1647 ) ;
#9671=CARTESIAN_POINT ( 'NONE',  ( -384.7236254841880623, 86.46752657155295196, -105.1769125859564014 ) ) ;
#9673=ORIENTED_EDGE ( 'NONE', *, *, #5229, .F. ) ;
#9677=FACE_OUTER_BOUND ( 'NONE', #10393, .T. ) ;
#9681=VERTEX_POINT ( 'NONE', #5258 ) ;
#9685=EDGE_LOOP ( 'NONE', ( #591, #10390 ) ) ;
#9688=EDGE_CURVE ( 'NONE', #3344, #7569, #5655, .T. ) ;
#9700=CARTESIAN_POINT ( 'NONE',  ( -180.0000000000000000, 24.00000000000001421, -126.4213562373082453 ) ) ;
#9702=EDGE_CURVE ( 'NONE', #7767, #1233, #7033, .T. ) ;
#9709=CARTESIAN_POINT ( 'NONE',  ( -270.0000000000000000, -9.213203435596478030, -126.4213562373076059 ) ) ;
#9710=VERTEX_POINT ( 'NONE', #8980 ) ;
#9712=CARTESIAN_POINT ( 'NONE',  ( -384.4692968731354199, 88.15998365774518675, -143.7178510142985886 ) ) ;
#9716=CARTESIAN_POINT ( 'NONE',  ( -240.0000000000000000, 24.00000000000000711, -126.4213562373078190 ) ) ;
#9718=SURFACE_SIDE_STYLE ('',( #5136 ) ) ;
#9719=AXIS2_PLACEMENT_3D ( 'NONE', #11258, #11125, #2650 ) ;
#9732=VERTEX_POINT ( 'NONE', #10841 ) ;
#9735=VECTOR ( 'NONE', #3489, 1000.000000000000000 ) ;
#9748=AXIS2_PLACEMENT_3D ( 'NONE', #10135, #4588, #8364 ) ;
#9753=DIRECTION ( 'NONE',  ( -0.000000000000000000, -0.000000000000000000, 1.000000000000000000 ) ) ;
#9756=DIRECTION ( 'NONE',  ( 0.000000000000000000, 0.000000000000000000, 1.000000000000000000 ) ) ;
#9758=DIRECTION ( 'NONE',  ( -1.000000000000000000, 0.000000000000000000, 0.000000000000000000 ) ) ;
#9760=AXIS2_PLACEMENT_3D ( 'NONE', #1451, #8201, #8987 ) ;
#9762=EDGE_CURVE ( 'NONE', #7569, #3344, #9608, .T. ) ;
#9769=FACE_BOUND ( 'NONE', #6868, .T. ) ;
#9774=DIRECTION ( 'NONE',  ( 0.000000000000000000, 1.000000000000000000, 0.000000000000000000 ) ) ;
#9775=DIRECTION ( 'NONE',  ( 3.061276722312011504E-17, -1.000000000000000000, 0.000000000000000000 ) ) ;
#9780=EDGE_CURVE ( 'NONE', #6370, #7586, #4274, .T. ) ;
#9786=DIRECTION ( 'NONE',  ( -8.163404592832030268E-17, 1.000000000000000000, -0.000000000000000000 ) ) ;
#9790=ORIENTED_EDGE ( 'NONE', *, *, #11514, .F. ) ;
#9798=CARTESIAN_POINT ( 'NONE',  ( -172.5000000000000000, 12.00000000000001421, -126.4213562373082453 ) ) ;
#9802=CARTESIAN_POINT ( 'NONE',  ( -374.6679438209018826, 88.82298366188321381, -95.70765607985160273 ) ) ;
#9803=ORIENTED_EDGE ( 'NONE', *, *, #7038, .T. ) ;
#9815=CARTESIAN_POINT ( 'NONE',  ( -379.5936447076720697, 62.72305949846725071, -119.2434292096965720 ) ) ;
#9821=CARTESIAN_POINT ( 'NONE',  ( -120.0000000000000000, 139.9999999999999716, -126.4213562373086575 ) ) ;
#9822=CARTESIAN_POINT ( 'NONE',  ( -375.0000000000000568, 82.00000000000093792, -94.68077099980381206 ) ) ;
#9824=EDGE_LOOP ( 'NONE', ( #3057, #124 ) ) ;
#9826=CARTESIAN_POINT ( 'NONE',  ( -384.1383856924539373, 74.17476869750447577, -143.0957938661287301 ) ) ;
#9830=CARTESIAN_POINT ( 'NONE',  ( -373.7989999032910191, 94.92607833831473840, -150.8034571341187586 ) ) ;
#9831=CARTESIAN_POINT ( 'NONE',  ( -67.50000000000000000, 152.0000000000000000, -126.4213562373090696 ) ) ;
#9832=CARTESIAN_POINT ( 'NONE',  ( -372.9400467759962226, 63.90640018081566609, -116.0698391000898511 ) ) ;
#9834=CYLINDRICAL_SURFACE ( 'NONE', #8463, 7.500000000000007105 ) ;
#9848=DIRECTION ( 'NONE',  ( -1.000000000000000000, 0.000000000000000000, 0.000000000000000000 ) ) ;
#9850=CARTESIAN_POINT ( 'NONE',  ( 1.414009460465297036E-14, -9.213203435596451385, -126.4213562373094959 ) ) ;
#9853=ORIENTED_EDGE ( 'NONE', *, *, #1799, .F. ) ;
#9859=DIRECTION ( 'NONE',  ( 0.000000000000000000, 0.000000000000000000, 1.000000000000000000 ) ) ;
#9864=DIRECTION ( 'NONE',  ( -8.163404592832030268E-17, 1.000000000000000000, -0.000000000000000000 ) ) ;
#9867=DIRECTION ( 'NONE',  ( -1.000000000000000000, 0.000000000000000000, 0.000000000000000000 ) ) ;
#9869=ORIENTED_EDGE ( 'NONE', *, *, #10556, .F. ) ;
#9872=CARTESIAN_POINT ( 'NONE',  ( -370.4401466759219375, 106.8513018378076822, -134.3428354745942102 ) ) ;
#9876=FACE_OUTER_BOUND ( 'NONE', #1309, .T. ) ;
#9877=CARTESIAN_POINT ( 'NONE',  ( -818.9962482452900758, 77.37998253221826417, -144.1405054422206717 ) ) ;
#9878=CARTESIAN_POINT ( 'NONE',  ( -828.7892213480602095, 79.32116703283860204, -104.8603099499564877 ) ) ;
#9880=CARTESIAN_POINT ( 'NONE',  ( -379.8598815838158202, 100.8093737612647658, -117.8752137794534320 ) ) ;
#9892=CARTESIAN_POINT ( 'NONE',  ( -382.3432055905735183, 68.36282604260088647, -139.3218746688176282 ) ) ;
#9894=DIRECTION ( 'NONE',  ( -1.000000000000000000, 0.000000000000000000, 0.000000000000000000 ) ) ;
#9897=ORIENTED_EDGE ( 'NONE', *, *, #5776, .F. ) ;
#9901=DIRECTION ( 'NONE',  ( 0.000000000000000000, 0.000000000000000000, 1.000000000000000000 ) ) ;
#9902=AXIS2_PLACEMENT_3D ( 'NONE', #7461, #6532, #5542 ) ;
#9905=CARTESIAN_POINT ( 'NONE',  ( -150.0000000000000000, -9.213203435596451385, -126.4213562373084301 ) ) ;
#9906=ORIENTED_EDGE ( 'NONE', *, *, #10601, .T. ) ;
#9914=CARTESIAN_POINT ( 'NONE',  ( -60.00000000000000000, 152.0000000000000000, -126.4213562373090696 ) ) ;
#9916=CARTESIAN_POINT ( 'NONE',  ( -305.0000000000000568, 24.00000000000000711, -89.68077099980384048 ) ) ;
#9919=CARTESIAN_POINT ( 'NONE',  ( -372.8632101103306695, 63.61025241748026815, -116.7299017350923833 ) ) ;
#9923=DIRECTION ( 'NONE',  ( -8.163404592832030268E-17, 1.000000000000000000, -0.000000000000000000 ) ) ;
#9934=CARTESIAN_POINT ( 'NONE',  ( -379.2306375576939672, 62.11345676130450499, -122.4830476075849788 ) ) ;
#9940=DIRECTION ( 'NONE',  ( 0.000000000000000000, 1.000000000000000000, -0.000000000000000000 ) ) ;
#9943=AXIS2_PLACEMENT_3D ( 'NONE', #4674, #5706, #10404 ) ;
#9952=AXIS2_PLACEMENT_3D ( 'NONE', #5940, #3157, #1073 ) ;
#9955=CARTESIAN_POINT ( 'NONE',  ( 35.00000000000000000, 152.0000000000000000, -89.68077099980384048 ) ) ;
#9958=CARTESIAN_POINT ( 'NONE',  ( -371.8264734514620500, 61.12950623280156037, -106.3821846224840755 ) ) ;
#9962=ORIENTED_EDGE ( 'NONE', *, *, #10971, .F. ) ;
#9969=FACE_OUTER_BOUND ( 'NONE', #11286, .T. ) ;
#9970=ORIENTED_EDGE ( 'NONE', *, *, #3945, .F. ) ;
#9972=AXIS2_PLACEMENT_3D ( 'NONE', #4294, #1565, #10221 ) ;
#9977=DIRECTION ( 'NONE',  ( -1.000000000000000000, 0.000000000000000000, 0.000000000000000000 ) ) ;
#9984=VERTEX_POINT ( 'NONE', #12210 ) ;
#9996=CARTESIAN_POINT ( 'NONE',  ( -820.5015944640188081, 74.92794535927947663, -143.3902763353420369 ) ) ;
#9999=EDGE_CURVE ( 'NONE', #6258, #6415, #1324, .T. ) ;
#10000=AXIS2_PLACEMENT_3D ( 'NONE', #652, #9923, #10850 ) ;
#10004=LINE ( 'NONE', #7225, #11013 ) ;
#10008=ORIENTED_EDGE ( 'NONE', *, *, #654, .F. ) ;
#10009=VECTOR ( 'NONE', #8839, 1000.000000000000000 ) ;
#10017=DIRECTION ( 'NONE',  ( -8.163404592832030268E-17, 1.000000000000000000, -0.000000000000000000 ) ) ;
#10025=EDGE_CURVE ( 'NONE', #6648, #6415, #8568, .T. ) ;
#10030=CARTESIAN_POINT ( 'NONE',  ( -370.0960371382928429, 56.26061672099882571, -130.5900565961996449 ) ) ;
#10034=CIRCLE ( 'NONE', #4717, 7.500000000000020428 ) ;
#10036=ORIENTED_EDGE ( 'NONE', *, *, #11359, .F. ) ;
#10039=CYLINDRICAL_SURFACE ( 'NONE', #10953, 7.500000000000007105 ) ;
#10041=AXIS2_PLACEMENT_3D ( 'NONE', #8845, #5010, #311 ) ;
#10044=DIRECTION ( 'NONE',  ( -1.000000000000000000, -3.061276722312011504E-17, -0.000000000000000000 ) ) ;
#10054=DIRECTION ( 'NONE',  ( 1.000000000000000000, 0.000000000000000000, 0.000000000000000000 ) ) ;
#10063=DIRECTION ( 'NONE',  ( -8.163404592832030268E-17, 1.000000000000000000, -0.000000000000000000 ) ) ;
#10068=DIRECTION ( 'NONE',  ( 1.000000000000000000, 0.000000000000000000, 0.000000000000000000 ) ) ;
#10069=CARTESIAN_POINT ( 'NONE',  ( -384.9422428523002964, 79.88598318847526514, -144.5779090198339532 ) ) ;
#10077=CARTESIAN_POINT ( 'NONE',  ( -240.0000000000000000, -9.213203435596478030, -126.4213562373078190 ) ) ;
#10083=VERTEX_POINT ( 'NONE', #3518 ) ;
#10089=CARTESIAN_POINT ( 'NONE',  ( -370.0632692633016063, 56.17797598930829395, -130.0988530496388478 ) ) ;
#10103=EDGE_LOOP ( 'NONE', ( #9465, #6477, #6070, #8555 ) ) ;
#10104=DIRECTION ( 'NONE',  ( -0.1214029594221266301, -0.3196865710829014384, -0.9397136892228434846 ) ) ;
#10106=DIRECTION ( 'NONE',  ( -8.163404592832031500E-17, 1.000000000000000000, 0.000000000000000000 ) ) ;
#10113=DIRECTION ( 'NONE',  ( -1.000000000000000000, 0.000000000000000000, 0.000000000000000000 ) ) ;
#10115=CARTESIAN_POINT ( 'NONE',  ( -827.1569714199375767, 74.92915896788937857, -105.9707980921569117 ) ) ;
#10119=CARTESIAN_POINT ( 'NONE',  ( -370.0557944711135292, 56.15912500487524994, -119.3740868421776327 ) ) ;
#10127=ORIENTED_EDGE ( 'NONE', *, *, #7473, .T. ) ;
#10130=CARTESIAN_POINT ( 'NONE',  ( -277.5000000000000000, -9.213203435596478030, -126.4213562373076059 ) ) ;
#10133=CARTESIAN_POINT ( 'NONE',  ( -379.1811916902539679, 101.9683303498903513, -125.9862397059319505 ) ) ;
#10135=CARTESIAN_POINT ( 'NONE',  ( -270.0000000000000000, 24.00000000000000711, -126.4213562373076059 ) ) ;
#10143=DIRECTION ( 'NONE',  ( 3.061276722312011504E-17, -1.000000000000000000, 0.000000000000000000 ) ) ;
#10148=CIRCLE ( 'NONE', #5790, 7.500000000000007994 ) ;
#10150=VERTEX_POINT ( 'NONE', #3759 ) ;
#10151=CARTESIAN_POINT ( 'NONE',  ( -380.0389975087255152, 63.50064549581343698, -132.3938157233661457 ) ) ;
#10152=CARTESIAN_POINT ( 'NONE',  ( -119.9999999999999858, -9.213203435596451385, -126.4213562373086575 ) ) ;
#10158=AXIS2_PLACEMENT_3D ( 'NONE', #6081, #5960, #8746 ) ;
#10159=CIRCLE ( 'NONE', #8778, 57.99999999999999289 ) ;
#10169=CARTESIAN_POINT ( 'NONE',  ( -819.0830098007990046, 80.28235241365167951, -144.6091609974195080 ) ) ;
#10180=CARTESIAN_POINT ( 'NONE',  ( -822.5144771496169369, 73.83866123373404378, -106.4215885538519615 ) ) ;
#10181=CARTESIAN_POINT ( 'NONE',  ( -824.1558762432716776, 73.68222816774701300, -142.8690915370043228 ) ) ;
#10190=DIRECTION ( 'NONE',  ( -1.000000000000000000, 0.000000000000000000, 0.000000000000000000 ) ) ;
#10197=FACE_OUTER_BOUND ( 'NONE', #7160, .T. ) ;
#10200=DIRECTION ( 'NONE',  ( -1.000000000000000000, 0.000000000000000000, 0.000000000000000000 ) ) ;
#10208=CARTESIAN_POINT ( 'NONE',  ( -383.2280749472602679, 93.16617163057104278, -141.2766522578266404 ) ) ;
#10211=VECTOR ( 'NONE', #2019, 1000.000000000000000 ) ;
#10214=ORIENTED_EDGE ( 'NONE', *, *, #542, .F. ) ;
#10219=CARTESIAN_POINT ( 'NONE',  ( -380.6759376891203601, 64.70238119921620523, -134.7256802324791636 ) ) ;
#10221=DIRECTION ( 'NONE',  ( 1.000000000000000000, 0.000000000000000000, 0.000000000000000000 ) ) ;
#10228=EDGE_CURVE ( 'NONE', #3468, #966, #9218, .T. ) ;
#10238=CARTESIAN_POINT ( 'NONE',  ( -370.0269349526453198, 107.9136251528400265, -119.7614542792374408 ) ) ;
#10246=CYLINDRICAL_SURFACE ( 'NONE', #9667, 5.000000000000004441 ) ;
#10252=CARTESIAN_POINT ( 'NONE',  ( -371.3024966496543584, 59.54890786220743593, -140.2366040927702784 ) ) ;
#10253=CARTESIAN_POINT ( 'NONE',  ( -371.6804198345414534, 103.3022927311476877, -107.1440333209211815 ) ) ;
#10260=AXIS2_PLACEMENT_3D ( 'NONE', #5123, #9753, #1298 ) ;
#10262=ORIENTED_EDGE ( 'NONE', *, *, #10556, .T. ) ;
#10267=CARTESIAN_POINT ( 'NONE',  ( -370.3453975627718933, 107.0997924316958176, -115.8836695100632994 ) ) ;
#10272=CARTESIAN_POINT ( 'NONE',  ( -383.3150907383348454, 92.89194869614372863, -141.4579310800400549 ) ) ;
#10278=ORIENTED_EDGE ( 'NONE', *, *, #5015, .T. ) ;
#10279=CARTESIAN_POINT ( 'NONE',  ( -372.1640597400288470, 62.26788882665526614, -144.4898947985778079 ) ) ;
#10283=DIRECTION ( 'NONE',  ( -8.163404592832030268E-17, 1.000000000000000000, -0.000000000000000000 ) ) ;
#10293=CARTESIAN_POINT ( 'NONE',  ( -150.0000000000000000, 139.9999999999999716, -126.4213562373084301 ) ) ;
#10294=ORIENTED_EDGE ( 'NONE', *, *, #7842, .T. ) ;
#10300=CYLINDRICAL_SURFACE ( 'NONE', #9902, 35.00000000000000000 ) ;
#10306=CARTESIAN_POINT ( 'NONE',  ( -374.2311861953731977, 71.64084721860098171, -152.2531916975700881 ) ) ;
#10307=CARTESIAN_POINT ( 'NONE',  ( -382.8879895414342514, 94.18609904179986358, -108.8085965833891890 ) ) ;
#10311=CARTESIAN_POINT ( 'NONE',  ( -180.0000000000000000, 151.9999999999999716, -126.4213562373082453 ) ) ;
#10312=EDGE_CURVE ( 'NONE', #3344, #9710, #3682, .T. ) ;
#10314=ORIENTED_EDGE ( 'NONE', *, *, #5082, .T. ) ;
#10318=CARTESIAN_POINT ( 'NONE',  ( -379.6261022631920810, 101.2176309556962082, -119.1318278414791507 ) ) ;
#10322=DIRECTION ( 'NONE',  ( 3.061276722312011504E-17, -1.000000000000000000, 0.000000000000000000 ) ) ;
#10325=CARTESIAN_POINT ( 'NONE',  ( -373.6516460492721308, 96.99228658101947076, -138.0176360913489191 ) ) ;
#10329=VECTOR ( 'NONE', #6405, 1000.000000000000000 ) ;
#10333=CARTESIAN_POINT ( 'NONE',  ( -375.0000000000000000, 81.99999999999995737, -89.68077099980384048 ) ) ;
#10335=FACE_BOUND ( 'NONE', #2047, .T. ) ;
#10338=CARTESIAN_POINT ( 'NONE',  ( -382.8924036478341009, 69.79657916374794979, -140.5797354247098099 ) ) ;
#10340=CARTESIAN_POINT ( 'NONE',  ( -374.2594319682045807, 70.51193190803552113, -108.2281409940259351 ) ) ;
#10343=VECTOR ( 'NONE', #9470, 1000.000000000000000 ) ;
#10348=DIRECTION ( 'NONE',  ( -8.163404592832030268E-17, 1.000000000000000000, -0.000000000000000000 ) ) ;
#10350=EDGE_LOOP ( 'NONE', ( #6944, #10214 ) ) ;
#10355=CARTESIAN_POINT ( 'NONE',  ( -373.4608161113892493, 96.60585252165465420, -99.74601397596084951 ) ) ;
#10356=ORIENTED_EDGE ( 'NONE', *, *, #2029, .F. ) ;
#10358=CARTESIAN_POINT ( 'NONE',  ( -37.49999999999999289, -9.213203435596451385, -126.4213562373092685 ) ) ;
#10361=ADVANCED_FACE ( 'NONE', ( #3401 ), #8019, .F. ) ;
#10363=FACE_BOUND ( 'NONE', #2938, .T. ) ;
#10368=AXIS2_PLACEMENT_3D ( 'NONE', #10805, #5929, #10744 ) ;
#10372=VERTEX_POINT ( 'NONE', #10792 ) ;
#10380=DIRECTION ( 'NONE',  ( -1.000000000000000000, 0.000000000000000000, 0.000000000000000000 ) ) ;
#10382=EDGE_CURVE ( 'NONE', #90, #2078, #5341, .T. ) ;
#10383=PRODUCT_DEFINITION_SHAPE ( 'NONE', 'NONE',  #9348 ) ;
#10387=DIRECTION ( 'NONE',  ( 1.000000000000000000, 0.000000000000000000, -0.000000000000000000 ) ) ;
#10390=ORIENTED_EDGE ( 'NONE', *, *, #5684, .T. ) ;
#10393=EDGE_LOOP ( 'NONE', ( #2805, #9341, #4450, #9326 ) ) ;
#10395=CARTESIAN_POINT ( 'NONE',  ( -382.4233354741761559, 68.57082533223261578, -139.5051951744822816 ) ) ;
#10397=CARTESIAN_POINT ( 'NONE',  ( -374.3220111056598967, 72.27247505761226876, -96.81229118638817965 ) ) ;
#10400=ORIENTED_EDGE ( 'NONE', *, *, #10450, .F. ) ;
#10404=DIRECTION ( 'NONE',  ( 1.000000000000000000, 0.000000000000000000, 0.000000000000000000 ) ) ;
#10408=CARTESIAN_POINT ( 'NONE',  ( -89.99999999999998579, 12.00000000000001421, -126.4213562373088564 ) ) ;
#10411=DIRECTION ( 'NONE',  ( -8.163404592832030268E-17, 1.000000000000000000, -0.000000000000000000 ) ) ;
#10413=CARTESIAN_POINT ( 'NONE',  ( -821.6112282492910026, 83.16771792585103640, -144.6470480974979864 ) ) ;
#10415=CARTESIAN_POINT ( 'NONE',  ( -369.9264633483897455, 108.1643382291179449, -122.0075474512173059 ) ) ;
#10419=AXIS2_PLACEMENT_3D ( 'NONE', #2123, #9775, #6993 ) ;
#10425=DIRECTION ( 'NONE',  ( 3.061276722312011504E-17, -1.000000000000000000, 0.000000000000000000 ) ) ;
#10430=CARTESIAN_POINT ( 'NONE',  ( -381.7638695068005745, 97.03891058473890041, -111.4316689550042270 ) ) ;
#10436=AXIS2_PLACEMENT_3D ( 'NONE', #6965, #2272, #4865 ) ;
#10444=CARTESIAN_POINT ( 'NONE',  ( -270.0000000000000000, 151.9999999999999716, -126.4213562373076059 ) ) ;
#10450=EDGE_CURVE ( 'NONE', #11532, #7797, #1736, .T. ) ;
#10454=AXIS2_PLACEMENT_3D ( 'NONE', #10444, #1062, #4819 ) ;
#10456=ORIENTED_EDGE ( 'NONE', *, *, #4516, .F. ) ;
#10457=ORIENTED_EDGE ( 'NONE', *, *, #7214, .T. ) ;
#10464=CARTESIAN_POINT ( 'NONE',  ( -384.3557402719069387, 75.23780925246066431, -143.5057597349512264 ) ) ;
#10466=CARTESIAN_POINT ( 'NONE',  ( -374.1438204953303739, 71.07787666357693013, -97.39646298909734412 ) ) ;
#10475=DIRECTION ( 'NONE',  ( -0.000000000000000000, -0.000000000000000000, -1.000000000000000000 ) ) ;
#10478=ORIENTED_EDGE ( 'NONE', *, *, #7595, .F. ) ;
#10480=CARTESIAN_POINT ( 'NONE',  ( -371.6737729595722044, 103.3297310517157115, -107.1558738098986083 ) ) ;
#10497=DIRECTION ( 'NONE',  ( -8.163404592832030268E-17, 1.000000000000000000, -0.000000000000000000 ) ) ;
#10504=B_SPLINE_CURVE_WITH_KNOTS ( 'NONE', 3,
 ( #2036, #5925, #3949, #6787, #10561, #10619, #1235, #8711, #4990, #227, #7781, #11557, #8770, #4078, #6911, #10677, #2216, #10740, #3431, #466, #9124, #11855, #5348, #1352, #4191, #3312, #6170, #5119, #11677, #11740, #8882, #2391, #7093, #5172, #9878, #3195, #7968, #10857 ),
 .UNSPECIFIED., .F., .F.,
 ( 4, 2, 2, 2, 2, 2, 2, 2, 2, 2, 2, 2, 2, 2, 2, 2, 2, 2, 4 ),
 ( 1.387778780781445676E-17, 0.0009791294386043965323, 0.001958258877208779187, 0.002937388315813161625, 0.003916517754417544496, 0.004895647193021926934, 0.005874776631626309371, 0.006364341350928661920, 0.006853906070231015335, 0.007833035508835389099, 0.008812164947439762863, 0.009791294386044136627, 0.01077042382464851039, 0.01174955326325288589, 0.01272868270185725792, 0.01370781214046163342, 0.01468694157906600545, 0.01517650629836820447, 0.01566607101767040003 ),
 .UNSPECIFIED. ) ;
#10508=ORIENTED_EDGE ( 'NONE', *, *, #8386, .F. ) ;
#10513=CYLINDRICAL_SURFACE ( 'NONE', #2318, 7.500000000000007105 ) ;
#10516=ADVANCED_FACE ( 'NONE', ( #4773 ), #10513, .F. ) ;
#10520=VERTEX_POINT ( 'NONE', #1193 ) ;
#10521=CARTESIAN_POINT ( 'NONE',  ( -374.9804624535815947, 84.15814354082083071, -144.5772115629533232 ) ) ;
#10523=EDGE_LOOP ( 'NONE', ( #619, #8956 ) ) ;
#10526=FACE_OUTER_BOUND ( 'NONE', #5413, .T. ) ;
#10527=AXIS2_PLACEMENT_3D ( 'NONE', #6775, #1046, #3071 ) ;
#10530=EDGE_CURVE ( 'NONE', #7375, #8861, #4092, .T. ) ;
#10536=ORIENTED_EDGE ( 'NONE', *, *, #342, .T. ) ;
#10541=FACE_OUTER_BOUND ( 'NONE', #2355, .T. ) ;
#10543=FACE_BOUND ( 'NONE', #7998, .T. ) ;
#10545=AXIS2_PLACEMENT_3D ( 'NONE', #3492, #5477, #11246 ) ;
#10549=CARTESIAN_POINT ( 'NONE',  ( -374.7821307776476942, 76.37722585493098393, -154.0118767560747699 ) ) ;
#10550=EDGE_CURVE ( 'NONE', #5774, #7370, #10725, .T. ) ;
#10553=EDGE_LOOP ( 'NONE', ( #1913, #9088 ) ) ;
#10556=EDGE_CURVE ( 'NONE', #1969, #6496, #1519, .T. ) ;
#10558=DIRECTION ( 'NONE',  ( -8.163404592832030268E-17, 1.000000000000000000, -0.000000000000000000 ) ) ;
#10561=CARTESIAN_POINT ( 'NONE',  ( -819.0811117622678239, 80.27710935352754973, -104.7528066153021626 ) ) ;
#10575=ORIENTED_EDGE ( 'NONE', *, *, #11671, .F. ) ;
#10581=CARTESIAN_POINT ( 'NONE',  ( -374.4965189541518953, 90.54923481422481757, -153.1149316092644597 ) ) ;
#10582=DIRECTION ( 'NONE',  ( 3.061276722312011504E-17, -1.000000000000000000, 0.000000000000000000 ) ) ;
#10583=CARTESIAN_POINT ( 'NONE',  ( -374.9791051857908997, 79.82954463378038668, -104.7910636793791355 ) ) ;
#10584=( LENGTH_UNIT ( ) NAMED_UNIT ( * ) SI_UNIT ( .MILLI., .METRE. ) );
#10589=CYLINDRICAL_SURFACE ( 'NONE', #4863, 7.500000000000007105 ) ;
#10593=EDGE_LOOP ( 'NONE', ( #6508, #4840, #5239, #6848 ) ) ;
#10595=CARTESIAN_POINT ( 'NONE',  ( -384.9968589487228883, 81.44061423874818217, -104.6863554354390118 ) ) ;
#10601=EDGE_CURVE ( 'NONE', #8983, #9452, #2716, .T. ) ;
#10603=DIRECTION ( 'NONE',  ( -8.163404592832030268E-17, 1.000000000000000000, -0.000000000000000000 ) ) ;
#10607=DIRECTION ( 'NONE',  ( 1.000000000000000000, 0.000000000000000000, 0.000000000000000000 ) ) ;
#10619=CARTESIAN_POINT ( 'NONE',  ( -819.3307005430665413, 80.88259174529672180, -104.7097040407755912 ) ) ;
#10622=CARTESIAN_POINT ( 'NONE',  ( -379.7973532621967934, 100.9195114153188797, -118.1876023976287087 ) ) ;
#10639=VECTOR ( 'NONE', #10702, 1000.000000000000000 ) ;
#10646=VERTEX_POINT ( 'NONE', #1573 ) ;
#10655=CARTESIAN_POINT ( 'NONE',  ( -383.8907576663274881, 90.90990570178517771, -106.7374497346880133 ) ) ;
#10673=CARTESIAN_POINT ( 'NONE',  ( 0.000000000000000000, 152.0000000000000000, -159.6807709998038547 ) ) ;
#10675=ORIENTED_EDGE ( 'NONE', *, *, #10382, .F. ) ;
#10677=CARTESIAN_POINT ( 'NONE',  ( -822.5306970061909624, 83.50573423571496789, -104.7374748144103336 ) ) ;
#10679=ADVANCED_FACE ( 'NONE', ( #7198 ), #12018, .F. ) ;
#10685=CARTESIAN_POINT ( 'NONE',  ( -305.0000000000000568, 81.99999999999995737, -89.68077099980384048 ) ) ;
#10698=CIRCLE ( 'NONE', #1044, 7.500000000000007105 ) ;
#10699=CARTESIAN_POINT ( 'NONE',  ( -374.5266264499630324, 90.13403016665176892, -153.2070368496501658 ) ) ;
#10702=DIRECTION ( 'NONE',  ( -0.000000000000000000, -0.000000000000000000, -1.000000000000000000 ) ) ;
#10711=CARTESIAN_POINT ( 'NONE',  ( -277.5000000000000000, -9.213203435596478030, -126.4213562373076059 ) ) ;
#10721=DIRECTION ( 'NONE',  ( 2.040851148208007875E-17, -1.000000000000000000, -0.000000000000000000 ) ) ;
#10725=LINE ( 'NONE', #10787, #3486 ) ;
#10727=EDGE_LOOP ( 'NONE', ( #10924, #563, #5996, #5336 ) ) ;
#10732=DIRECTION ( 'NONE',  ( 0.000000000000000000, 0.000000000000000000, 1.000000000000000000 ) ) ;
#10737=VECTOR ( 'NONE', #9638, 1000.000000000000000 ) ;
#10740=CARTESIAN_POINT ( 'NONE',  ( -823.1752771847263830, 83.64233931405162537, -104.7482132693508419 ) ) ;
#10741=DIRECTION ( 'NONE',  ( 1.000000000000000000, 1.486905836551548832E-16, -0.000000000000000000 ) ) ;
#10742=CARTESIAN_POINT ( 'NONE',  ( -373.0282128842003431, 99.74530980265677726, -115.3648426268730276 ) ) ;
#10744=DIRECTION ( 'NONE',  ( 1.000000000000000000, 3.061276722312011504E-17, 0.000000000000000000 ) ) ;
#10746=DIRECTION ( 'NONE',  ( -1.000000000000000000, 0.000000000000000000, 0.000000000000000000 ) ) ;
#10749=VECTOR ( 'NONE', #53, 1000.000000000000000 ) ;
#10750=DIRECTION ( 'NONE',  ( 0.000000000000000000, 0.000000000000000000, 1.000000000000000000 ) ) ;
#10752=DIRECTION ( 'NONE',  ( -1.000000000000000000, 0.000000000000000000, 0.000000000000000000 ) ) ;
#10753=ADVANCED_FACE ( 'NONE', ( #6822 ), #1022, .F. ) ;
#10756=CIRCLE ( 'NONE', #8005, 7.500000000000007105 ) ;
#10757=CARTESIAN_POINT ( 'NONE',  ( -380.1407962618786200, 63.69369713673138023, -132.7567463350160892 ) ) ;
#10759=CARTESIAN_POINT ( 'NONE',  ( -374.1268486318114128, 93.09154424955353591, -151.9171935354461596 ) ) ;
#10761=CARTESIAN_POINT ( 'NONE',  ( -373.1046688609678768, 64.56459520230322369, -114.7895357036745025 ) ) ;
#10762=FACE_OUTER_BOUND ( 'NONE', #6813, .T. ) ;
#10773=DIRECTION ( 'NONE',  ( -8.163404592832030268E-17, 1.000000000000000000, -0.000000000000000000 ) ) ;
#10778=ORIENTED_EDGE ( 'NONE', *, *, #1316, .T. ) ;
#10785=ADVANCED_FACE ( 'NONE', ( #5322, #4404, #5813, #2052, #3724, #2800, #7678, #6570, #1011, #10335, #1935 ), #5640, .F. ) ;
#10787=CARTESIAN_POINT ( 'NONE',  ( -82.49999999999997158, -9.213203435596451385, -126.4213562373088564 ) ) ;
#10791=VERTEX_POINT ( 'NONE', #11325 ) ;
#10792=CARTESIAN_POINT ( 'NONE',  ( -22.49999999999999289, 152.0000000000000000, -126.4213562373092685 ) ) ;
#10795=DIRECTION ( 'NONE',  ( -8.163404592832031500E-17, 1.000000000000000000, 0.000000000000000000 ) ) ;
#10800=CARTESIAN_POINT ( 'NONE',  ( -818.8285638327206470, 78.67432280806529832, -144.4023295390026931 ) ) ;
#10805=CARTESIAN_POINT ( 'NONE',  ( -305.0000000000000568, 24.00000000000000711, -89.68077099980384048 ) ) ;
#10807=CARTESIAN_POINT ( 'NONE',  ( -270.0000000000000000, -9.213203435596478030, -126.4213562373076059 ) ) ;
#10810=CARTESIAN_POINT ( 'NONE',  ( -375.0000000000001705, 81.27848041085138675, -94.68077099980376943 ) ) ;
#10817=EDGE_CURVE ( 'NONE', #1708, #3156, #7443, .T. ) ;
#10818=DIRECTION ( 'NONE',  ( 3.061276722312011504E-17, -1.000000000000000000, 0.000000000000000000 ) ) ;
#10820=CARTESIAN_POINT ( 'NONE',  ( -7.500000000000007105, 152.0000000000000000, -126.4213562373094959 ) ) ;
#10821=EDGE_CURVE ( 'NONE', #11612, #7375, #12198, .T. ) ;
#10838=FACE_OUTER_BOUND ( 'NONE', #5087, .T. ) ;
#10841=CARTESIAN_POINT ( 'NONE',  ( -157.5000000000000000, 152.0000000000000000, -126.4213562373084301 ) ) ;
#10845=CARTESIAN_POINT ( 'NONE',  ( -374.8742850566777634, 86.27977464002199781, -95.06579166030898875 ) ) ;
#10850=DIRECTION ( 'NONE',  ( -1.000000000000000000, 0.000000000000000000, 0.000000000000000000 ) ) ;
#10857=CARTESIAN_POINT ( 'NONE',  ( -828.8285638327206470, 78.67432280806529832, -104.9592124606049879 ) ) ;
#10858=CARTESIAN_POINT ( 'NONE',  ( -379.2722913866882664, 62.18251865808234413, -121.9290846803070849 ) ) ;
#10864=DIRECTION ( 'NONE',  ( -8.163404592832030268E-17, 1.000000000000000000, -0.000000000000000000 ) ) ;
#10870=CARTESIAN_POINT ( 'NONE',  ( -384.2568156453588131, 74.72561187594924093, -143.3202744651779312 ) ) ;
#10874=CARTESIAN_POINT ( 'NONE',  ( -370.5975445210319776, 106.4368310733506746, -135.7352130142525937 ) ) ;
#10889=DIRECTION ( 'NONE',  ( -8.163404592832030268E-17, 1.000000000000000000, -0.000000000000000000 ) ) ;
#10900=CARTESIAN_POINT ( 'NONE',  ( -172.5000000000000000, -9.213203435596478030, -126.4213562373082453 ) ) ;
#10901=CARTESIAN_POINT ( 'NONE',  ( -375.0000000000000568, 82.00000000000093792, -94.68077099980381206 ) ) ;
#10904=DIRECTION ( 'NONE',  ( 0.000000000000000000, 0.000000000000000000, 1.000000000000000000 ) ) ;
#10914=CARTESIAN_POINT ( 'NONE',  ( -142.5000000000000000, 12.00000000000001421, -126.4213562373084301 ) ) ;
#10916=DIRECTION ( 'NONE',  ( 1.000000000000000000, 0.000000000000000000, 0.000000000000000000 ) ) ;
#10921=EDGE_CURVE ( 'NONE', #8735, #11690, #8960, .T. ) ;
#10924=ORIENTED_EDGE ( 'NONE', *, *, #6406, .T. ) ;
#10928=EDGE_CURVE ( 'NONE', #8918, #1810, #7871, .T. ) ;
#10939=LINE ( 'NONE', #2526, #1461 ) ;
#10940=CARTESIAN_POINT ( 'NONE',  ( -372.4159675733355357, 102.0139246166868077, -124.6604683294675766 ) ) ;
#10947=CARTESIAN_POINT ( 'NONE',  ( 0.000000000000000000, 24.00000000000001776, -124.6807709998038405 ) ) ;
#10948=CARTESIAN_POINT ( 'NONE',  ( -157.5000000000000000, 24.00000000000001421, -126.4213562373084301 ) ) ;
#10949=ORIENTED_EDGE ( 'NONE', *, *, #10921, .F. ) ;
#10953=AXIS2_PLACEMENT_3D ( 'NONE', #1568, #2375, #3732 ) ;
#10957=CARTESIAN_POINT ( 'NONE',  ( -372.6561862956065738, 62.83025961264725368, -118.7578631316695237 ) ) ;
#10963=LINE ( 'NONE', #3233, #4445 ) ;
#10970=CARTESIAN_POINT ( 'NONE',  ( -277.5000000000000000, 139.9999999999999716, -126.4213562373076059 ) ) ;
#10971=EDGE_CURVE ( 'NONE', #6153, #6627, #10159, .T. ) ;
#10974=DIRECTION ( 'NONE',  ( -0.000000000000000000, 1.000000000000000000, -0.000000000000000000 ) ) ;
#10982=EDGE_CURVE ( 'NONE', #9219, #11532, #2995, .T. ) ;
#10987=ORIENTED_EDGE ( 'NONE', *, *, #1799, .T. ) ;
#10992=CARTESIAN_POINT ( 'NONE',  ( -7.499999999999998224, 24.00000000000001421, -126.4213562373094959 ) ) ;
#10999=CARTESIAN_POINT ( 'NONE',  ( -379.1619848709566440, 61.99999999999992184, -124.6807709998039542 ) ) ;
#11003=CARTESIAN_POINT ( 'NONE',  ( -277.5000000000000000, 12.00000000000001066, -126.4213562373076059 ) ) ;
#11013=VECTOR ( 'NONE', #2642, 1000.000000000000000 ) ;
#11016=CARTESIAN_POINT ( 'NONE',  ( -369.8688452567520812, 55.69319535620513051, -124.6859973355406197 ) ) ;
#11019=CIRCLE ( 'NONE', #5884, 7.500000000000020428 ) ;
#11022=AXIS2_PLACEMENT_3D ( 'NONE', #10807, #1358, #11681 ) ;
#11025=EDGE_CURVE ( 'NONE', #6366, #9074, #7394, .T. ) ;
#11031=ORIENTED_EDGE ( 'NONE', *, *, #1418, .T. ) ;
#11037=DIRECTION ( 'NONE',  ( 0.000000000000000000, 0.000000000000000000, 1.000000000000000000 ) ) ;
#11040=CIRCLE ( 'NONE', #6114, 7.500000000000007105 ) ;
#11043=CARTESIAN_POINT ( 'NONE',  ( -828.1717276517521213, 76.17609097696448828, -105.5454165443656507 ) ) ;
#11045=CARTESIAN_POINT ( 'NONE',  ( -828.3261744505556408, 76.46613818254095918, -143.9024326026597294 ) ) ;
#11047=ORIENTED_EDGE ( 'NONE', *, *, #7129, .F. ) ;
#11053=CARTESIAN_POINT ( 'NONE',  ( -210.0000000000000000, 24.00000000000000711, -126.4213562373080180 ) ) ;
#11062=CARTESIAN_POINT ( 'NONE',  ( -127.4999999999999716, 12.00000000000001421, -126.4213562373086575 ) ) ;
#11064=CARTESIAN_POINT ( 'NONE',  ( -369.9371856203899824, 108.1376465818777177, -127.6226701653134796 ) ) ;
#11065=EDGE_CURVE ( 'NONE', #966, #3468, #6207, .T. ) ;
#11073=CARTESIAN_POINT ( 'NONE',  ( -89.99999999999998579, 24.00000000000001421, -126.4213562373088564 ) ) ;
#11077=FACE_OUTER_BOUND ( 'NONE', #698, .T. ) ;
#11080=ORIENTED_EDGE ( 'NONE', *, *, #3520, .T. ) ;
#11082=CARTESIAN_POINT ( 'NONE',  ( -379.5247776001849616, 62.60840276516706382, -129.5872912034053286 ) ) ;
#11084=VERTEX_POINT ( 'NONE', #3064 ) ;
#11085=CYLINDRICAL_SURFACE ( 'NONE', #503, 7.499999999999992895 ) ;
#11096=CIRCLE ( 'NONE', #3789, 7.500000000000007105 ) ;
#11098=CARTESIAN_POINT ( 'NONE',  ( -828.8285638327206470, 78.67432280806529832, -144.4023295390027215 ) ) ;
#11107=CIRCLE ( 'NONE', #2222, 7.500000000000020428 ) ;
#11108=CARTESIAN_POINT ( 'NONE',  ( -826.0807747705194970, 74.19805998537496805, -106.2647609865421430 ) ) ;
#11110=DIRECTION ( 'NONE',  ( -8.163404592832031500E-17, 1.000000000000000000, -0.000000000000000000 ) ) ;
#11111=EDGE_LOOP ( 'NONE', ( #4898, #8676, #4111, #4617 ) ) ;
#11112=ORIENTED_EDGE ( 'NONE', *, *, #2079, .F. ) ;
#11113=CARTESIAN_POINT ( 'NONE',  ( -371.0428122657798440, 58.79643506041531964, -138.7203693468078427 ) ) ;
#11118=ADVANCED_FACE ( 'NONE', ( #10541 ), #6833, .F. ) ;
#11121=CARTESIAN_POINT ( 'NONE',  ( -372.9440792399824431, 65.15140800462232562, -101.6629770149452128 ) ) ;
#11123=VECTOR ( 'NONE', #3618, 1000.000000000000000 ) ;
#11125=DIRECTION ( 'NONE',  ( 2.040851148208007875E-17, -1.000000000000000000, -0.000000000000000000 ) ) ;
#11128=CARTESIAN_POINT ( 'NONE',  ( -369.8859280133687548, 108.2643723699462726, -124.6535011946241127 ) ) ;
#11134=DIRECTION ( 'NONE',  ( -1.000000000000000000, 0.000000000000000000, 0.000000000000000000 ) ) ;
#11135=AXIS2_PLACEMENT_3D ( 'NONE', #8391, #4788, #5454 ) ;
#11136=ADVANCED_FACE ( 'NONE', ( #8810 ), #2142, .F. ) ;
#11137=ORIENTED_EDGE ( 'NONE', *, *, #9762, .T. ) ;
#11139=ADVANCED_FACE ( 'NONE', ( #9677 ), #8572, .F. ) ;
#11140=VERTEX_POINT ( 'NONE', #6711 ) ;
#11148=ORIENTED_EDGE ( 'NONE', *, *, #3586, .F. ) ;
#11150=CARTESIAN_POINT ( 'NONE',  ( -373.4729226597870024, 66.15791503844970123, -136.9867814967885238 ) ) ;
#11153=CYLINDRICAL_SURFACE ( 'NONE', #4444, 7.500000000000007105 ) ;
#11160=CARTESIAN_POINT ( 'NONE',  ( -379.1619848709566440, 61.99999999999992184, -124.6807709998039542 ) ) ;
#11164=ORIENTED_EDGE ( 'NONE', *, *, #10550, .F. ) ;
#11167=CARTESIAN_POINT ( 'NONE',  ( -370.2377583643716434, 107.3781601596609221, -116.9922470894815945 ) ) ;
#11174=ADVANCED_FACE ( 'NONE', ( #149 ), #3177, .F. ) ;
#11175=CARTESIAN_POINT ( 'NONE',  ( -29.99999999999998934, 24.00000000000001421, -126.4213562373092685 ) ) ;
#11177=CARTESIAN_POINT ( 'NONE',  ( -828.8285638327206470, 78.67432280806529832, -104.9592124606049879 ) ) ;
#11179=CARTESIAN_POINT ( 'NONE',  ( -828.8285638327209881, 78.51036871773257531, -144.3746817048997855 ) ) ;
#11182=CARTESIAN_POINT ( 'NONE',  ( -370.2814337190545189, 56.73344489815470126, -132.8949611453235491 ) ) ;
#11183=CARTESIAN_POINT ( 'NONE',  ( -371.4445559945335162, 104.0267551742128660, -108.3548430067642698 ) ) ;
#11185=AXIS2_PLACEMENT_3D ( 'NONE', #6430, #5306, #10200 ) ;
#11192=ORIENTED_EDGE ( 'NONE', *, *, #10025, .F. ) ;
#11194=ORIENTED_EDGE ( 'NONE', *, *, #1984, .F. ) ;
#11200=CARTESIAN_POINT ( 'NONE',  ( -370.2978394803209881, 107.2231406293463749, -116.3573562623202235 ) ) ;
#11201=DIRECTION ( 'NONE',  ( -1.000000000000000000, -8.163404592832031500E-17, 0.000000000000000000 ) ) ;
#11205=CARTESIAN_POINT ( 'NONE',  ( -382.9619892260665210, 93.96448540389030768, -140.7106330510814303 ) ) ;
#11206=VERTEX_POINT ( 'NONE', #7703 ) ;
#11211=EDGE_CURVE ( 'NONE', #11690, #8735, #2266, .T. ) ;
#11214=AXIS2_PLACEMENT_3D ( 'NONE', #9700, #7975, #8939 ) ;
#11218=CARTESIAN_POINT ( 'NONE',  ( -379.4788071961805827, 62.53013482031470716, -129.2670437572034245 ) ) ;
#11229=CARTESIAN_POINT ( 'NONE',  ( -379.4314023685043935, 101.5510643398535393, -129.0327286575446806 ) ) ;
#11231=VERTEX_POINT ( 'NONE', #8979 ) ;
#11240=CARTESIAN_POINT ( 'NONE',  ( -112.4999999999999716, 12.00000000000001421, -126.4213562373086575 ) ) ;
#11242=AXIS2_PLACEMENT_3D ( 'NONE', #9000, #5984, #8883 ) ;
#11246=DIRECTION ( 'NONE',  ( -1.000000000000000000, 0.000000000000000000, 0.000000000000000000 ) ) ;
#11251=ORIENTED_EDGE ( 'NONE', *, *, #6820, .T. ) ;
#11255=ORIENTED_EDGE ( 'NONE', *, *, #4496, .T. ) ;
#11258=CARTESIAN_POINT ( 'NONE',  ( -29.99999999999998579, 12.00000000000001776, -126.4213562373092685 ) ) ;
#11264=CARTESIAN_POINT ( 'NONE',  ( -373.4495655788976478, 96.65560026510921432, -149.5745928868048793 ) ) ;
#11272=CARTESIAN_POINT ( 'NONE',  ( -372.7454185398722757, 64.37420824858371304, -146.9174072618011451 ) ) ;
#11273=CYLINDRICAL_SURFACE ( 'NONE', #1435, 7.500000000000007105 ) ;
#11274=CARTESIAN_POINT ( 'NONE',  ( -373.0607415668539488, 65.63369181740749525, -101.2204817476631149 ) ) ;
#11275=DIRECTION ( 'NONE',  ( 0.000000000000000000, 0.000000000000000000, 1.000000000000000000 ) ) ;
#11283=VERTEX_POINT ( 'NONE', #1441 ) ;
#11284=CARTESIAN_POINT ( 'NONE',  ( -828.1678681009874481, 81.16376924194455000, -144.6638077543058785 ) ) ;
#11286=EDGE_LOOP ( 'NONE', ( #7330, #2781, #11408, #3631 ) ) ;
#11296=CARTESIAN_POINT ( 'NONE',  ( -373.4631759638398307, 96.59209656397271715, -99.73825686774256383 ) ) ;
#11315=CARTESIAN_POINT ( 'NONE',  ( -374.3697334861134323, 92.69272124223820697, -141.6596876525885307 ) ) ;
#11316=ORIENTED_EDGE ( 'NONE', *, *, #9688, .F. ) ;
#11320=ORIENTED_EDGE ( 'NONE', *, *, #11065, .F. ) ;
#11325=CARTESIAN_POINT ( 'NONE',  ( -818.8285638327206470, 78.67432280806529832, -144.4023295390026931 ) ) ;
#11329=CARTESIAN_POINT ( 'NONE',  ( -374.9564170155092597, 84.61582091868922362, -154.5477554669674305 ) ) ;
#11340=CARTESIAN_POINT ( 'NONE',  ( -827.6030183929041186, 81.96987526947627600, -144.6820941065182069 ) ) ;
#11341=AXIS2_PLACEMENT_3D ( 'NONE', #648, #10104, #1637 ) ;
#11343=AXIS2_PLACEMENT_3D ( 'NONE', #10408, #5711, #8560 ) ;
#11348=DIRECTION ( 'NONE',  ( 1.000000000000000000, 2.040851148208007875E-17, 0.000000000000000000 ) ) ;
#11355=DIRECTION ( 'NONE',  ( -8.163404592832030268E-17, 1.000000000000000000, -0.000000000000000000 ) ) ;
#11358=CARTESIAN_POINT ( 'NONE',  ( -374.5812891589289961, 89.65635038802255963, -95.98092888736175610 ) ) ;
#11359=EDGE_CURVE ( 'NONE', #3156, #7498, #10963, .T. ) ;
#11363=CARTESIAN_POINT ( 'NONE',  ( -363.0000000000000568, 81.99999999999995737, -89.68077099980384048 ) ) ;
#11369=CARTESIAN_POINT ( 'NONE',  ( -828.8285638327206470, 78.67432280806529832, -264.6807709998040536 ) ) ;
#11376=CARTESIAN_POINT ( 'NONE',  ( -374.2771194692035692, 92.15366326334435598, -152.4146676682642010 ) ) ;
#11385=CARTESIAN_POINT ( 'NONE',  ( -383.1580143002730665, 93.38886992431909562, -141.1315691075368193 ) ) ;
#11386=DIRECTION ( 'NONE',  ( 0.000000000000000000, 0.000000000000000000, 1.000000000000000000 ) ) ;
#11389=CARTESIAN_POINT ( 'NONE',  ( -384.9501908748870278, 83.99300641423289449, -144.5920939778981733 ) ) ;
#11390=CARTESIAN_POINT ( 'NONE',  ( -305.0000000000000568, 24.00000000000000711, -89.68077099980384048 ) ) ;
#11391=CARTESIAN_POINT ( 'NONE',  ( -374.7441414241753819, 75.96258608733518258, -95.46849099916960313 ) ) ;
#11397=CARTESIAN_POINT ( 'NONE',  ( -29.99999999999998579, -9.213203435596451385, -126.4213562373092685 ) ) ;
#11403=CARTESIAN_POINT ( 'NONE',  ( -381.8446789258243825, 67.15007266234491112, -111.2347306979282848 ) ) ;
#11408=ORIENTED_EDGE ( 'NONE', *, *, #2215, .F. ) ;
#11414=PLANE ( 'NONE',  #7899 ) ;
#11419=CARTESIAN_POINT ( 'NONE',  ( -382.7045174276864259, 94.69426221061047499, -109.2122950466990829 ) ) ;
#11420=VERTEX_POINT ( 'NONE', #5150 ) ;
#11424=CARTESIAN_POINT ( 'NONE',  ( -180.0000000000000000, -9.213203435596478030, -126.4213562373082453 ) ) ;
#11425=AXIS2_PLACEMENT_3D ( 'NONE', #10947, #9774, #8961 ) ;
#11426=ADVANCED_FACE ( 'NONE', ( #10838 ), #10039, .F. ) ;
#11430=CYLINDRICAL_SURFACE ( 'NONE', #8720, 7.500000000000007105 ) ;
#11433=LINE ( 'NONE', #2967, #11930 ) ;
#11437=CARTESIAN_POINT ( 'NONE',  ( -379.7887390581964837, 100.9343252097582422, -131.1221473163307678 ) ) ;
#11448=CARTESIAN_POINT ( 'NONE',  ( -305.0000000000000568, 12.00000000000001066, -89.68077099980384048 ) ) ;
#11451=CARTESIAN_POINT ( 'NONE',  ( -374.9532740794444408, 85.24015211620390176, -144.4367336822883203 ) ) ;
#11453=CARTESIAN_POINT ( 'NONE',  ( -372.4851915888308440, 63.39452537575517255, -103.4953678669831731 ) ) ;
#11457=ORIENTED_EDGE ( 'NONE', *, *, #903, .F. ) ;
#11461=EDGE_CURVE ( 'NONE', #8369, #6191, #3422, .T. ) ;
#11464=DIRECTION ( 'NONE',  ( 1.000000000000000000, 0.000000000000000000, 0.000000000000000000 ) ) ;
#11466=CARTESIAN_POINT ( 'NONE',  ( -383.3096726399348881, 92.91657833282617673, -107.9127011693687592 ) ) ;
#11467=ORIENTED_EDGE ( 'NONE', *, *, #1316, .F. ) ;
#11475=CARTESIAN_POINT ( 'NONE',  ( -52.49999999999997868, -9.213203435596451385, -126.4213562373090696 ) ) ;
#11476=DIRECTION ( 'NONE',  ( 1.000000000000000000, 0.000000000000000000, 0.000000000000000000 ) ) ;
#11483=CARTESIAN_POINT ( 'NONE',  ( -374.9244159347675236, 86.03385731159455929, -105.0706672234830279 ) ) ;
#11492=DIRECTION ( 'NONE',  ( -8.163404592832030268E-17, 1.000000000000000000, -0.000000000000000000 ) ) ;
#11503=DIRECTION ( 'NONE',  ( -1.000000000000000000, 0.000000000000000000, 0.000000000000000000 ) ) ;
#11509=ORIENTED_EDGE ( 'NONE', *, *, #8944, .T. ) ;
#11510=ADVANCED_FACE ( 'NONE', ( #606 ), #8351, .F. ) ;
#11511=CARTESIAN_POINT ( 'NONE',  ( -384.9881694512860122, 81.02463022630767853, -144.6597318544169468 ) ) ;
#11513=CARTESIAN_POINT ( 'NONE',  ( -372.3192185535621661, 62.80464693345950877, -104.1946045324745143 ) ) ;
#11514=EDGE_CURVE ( 'NONE', #7370, #10150, #9176, .T. ) ;
#11519=VERTEX_POINT ( 'NONE', #7165 ) ;
#11526=CARTESIAN_POINT ( 'NONE',  ( -380.8706770098667675, 65.08321416438575113, -113.9963688427722133 ) ) ;
#11532=VERTEX_POINT ( 'NONE', #10992 ) ;
#11534=VECTOR ( 'NONE', #7384, 1000.000000000000000 ) ;
#11536=LINE ( 'NONE', #6832, #5096 ) ;
#11542=CARTESIAN_POINT ( 'NONE',  ( -305.0000000000000568, 81.99999999999995737, -159.6807709998038547 ) ) ;
#11550=EDGE_CURVE ( 'NONE', #8380, #7767, #6652, .T. ) ;
#11551=ORIENTED_EDGE ( 'NONE', *, *, #1229, .F. ) ;
#11557=CARTESIAN_POINT ( 'NONE',  ( -821.3208927675245832, 83.01261617297987527, -104.7055743826751524 ) ) ;
#11564=( NAMED_UNIT ( * ) SI_UNIT ( $, .STERADIAN. ) SOLID_ANGLE_UNIT ( ) );
#11571=EDGE_LOOP ( 'NONE', ( #380, #2522, #5137, #8018 ) ) ;
#11572=CARTESIAN_POINT ( 'NONE',  ( -382.1799076831810567, 96.06408218159914725, -138.9468483416044080 ) ) ;
#11577=SURFACE_STYLE_USAGE ( .BOTH. , #9718 ) ;
#11586=EDGE_CURVE ( 'NONE', #9164, #3075, #8097, .T. ) ;
#11593=CARTESIAN_POINT ( 'NONE',  ( -382.9953213592942802, 93.87473434840769926, -108.5770281898287237 ) ) ;
#11612=VERTEX_POINT ( 'NONE', #3386 ) ;
#11622=ADVANCED_FACE ( 'NONE', ( #11869 ), #1802, .F. ) ;
#11629=CARTESIAN_POINT ( 'NONE',  ( -370.4401466759219375, 106.8513018378076964, -134.3428354745942102 ) ) ;
#11634=CARTESIAN_POINT ( 'NONE',  ( -112.4999999999999716, -9.213203435596451385, -126.4213562373086575 ) ) ;
#11635=EDGE_LOOP ( 'NONE', ( #1204, #3229, #11255, #2305 ) ) ;
#11638=CARTESIAN_POINT ( 'NONE',  ( -384.9187498600809931, 84.67419646485878104, -144.5370176048736539 ) ) ;
#11641=CARTESIAN_POINT ( 'NONE',  ( -374.6737801889016168, 88.75927878213079225, -153.6720828349020849 ) ) ;
#11650=CARTESIAN_POINT ( 'NONE',  ( -379.3727436124818269, 62.35000097320466494, -120.7242238939077339 ) ) ;
#11654=EDGE_LOOP ( 'NONE', ( #3340, #8182 ) ) ;
#11665=ORIENTED_EDGE ( 'NONE', *, *, #2317, .F. ) ;
#11671=EDGE_CURVE ( 'NONE', #6366, #3468, #9279, .T. ) ;
#11675=LINE ( 'NONE', #5920, #1760 ) ;
#11676=CARTESIAN_POINT ( 'NONE',  ( -37.49999999999999289, -9.213203435596451385, -126.4213562373092685 ) ) ;
#11677=CARTESIAN_POINT ( 'NONE',  ( -827.8090925714915329, 81.71768170412174470, -104.6809152895176851 ) ) ;
#11678=CARTESIAN_POINT ( 'NONE',  ( -365.0000000000000568, 61.99999999999992895, -124.6807709998038405 ) ) ;
#11681=DIRECTION ( 'NONE',  ( -1.000000000000000000, 0.000000000000000000, 0.000000000000000000 ) ) ;
#11690=VERTEX_POINT ( 'NONE', #11003 ) ;
#11693=CARTESIAN_POINT ( 'NONE',  ( -379.2267265911639811, 62.10569044149951168, -127.0610581819159250 ) ) ;
#11697=CARTESIAN_POINT ( 'NONE',  ( -374.7703100637729676, 87.70944966426152689, -153.9741766301830239 ) ) ;
#11699=CARTESIAN_POINT ( 'NONE',  ( -373.1928135428791506, 64.92830709045685467, -114.1675738471262633 ) ) ;
#11701=CARTESIAN_POINT ( 'NONE',  ( -262.5000000000000000, 24.00000000000000711, -126.4213562373076059 ) ) ;
#11708=EDGE_LOOP ( 'NONE', ( #10457, #4860 ) ) ;
#11712=DIRECTION ( 'NONE',  ( -1.000000000000000000, 0.000000000000000000, 0.000000000000000000 ) ) ;
#11715=ORIENTED_EDGE ( 'NONE', *, *, #1984, .T. ) ;
#11716=ORIENTED_EDGE ( 'NONE', *, *, #2772, .F. ) ;
#11724=CIRCLE ( 'NONE', #6981, 7.500000000000007105 ) ;
#11728=DIRECTION ( 'NONE',  ( 0.000000000000000000, 1.000000000000000000, -0.000000000000000000 ) ) ;
#11740=CARTESIAN_POINT ( 'NONE',  ( -828.1711263241217011, 81.17408148015023528, -104.6959820179050951 ) ) ;
#11755=EDGE_CURVE ( 'NONE', #192, #5774, #10756, .T. ) ;
#11759=CARTESIAN_POINT ( 'NONE',  ( -372.3000261716298382, 101.2597060943377301, -145.0788949275182347 ) ) ;
#11761=CARTESIAN_POINT ( 'NONE',  ( -371.0605248364101953, 58.84368270872280249, -110.5171750812754965 ) ) ;
#11772=ORIENTED_EDGE ( 'NONE', *, *, #4565, .F. ) ;
#11773=B_SPLINE_CURVE_WITH_KNOTS ( 'NONE', 3,
 ( #11177, #922, #3490, #4695, #12231, #658, #11043, #12034, #6340, #10115, #3750, #3547, #11108, #2769, #7523, #3612, #2630, #6285, #9251, #861, #5346, #10180, #1717, #4562, #5476, #794, #8339, #4629, #12103, #8409, #12171, #7464, #3688, #3012, #3997, #6593 ),
 .UNSPECIFIED., .F., .F.,
 ( 4, 2, 2, 2, 2, 2, 2, 2, 2, 2, 2, 2, 2, 2, 2, 2, 2, 4 ),
 ( 0.01566607101767040003, 0.01666400919013317009, 0.01766194736259593667, 0.01865988553505870673, 0.01965782370752147332, 0.02065576187998424337, 0.02165370005244700996, 0.02215266913867839152, 0.02265163822490976961, 0.02364957639737220313, 0.02464751456983464012, 0.02564545274229707017, 0.02664339091475950369, 0.02764132908722193721, 0.02863926725968437073, 0.02963720543214680425, 0.03063514360460923777, 0.03163308177707167129 ),
 .UNSPECIFIED. ) ;
#11774=ORIENTED_EDGE ( 'NONE', *, *, #2675, .T. ) ;
#11776=CARTESIAN_POINT ( 'NONE',  ( -210.0000000000000000, 12.00000000000001421, -126.4213562373080180 ) ) ;
#11779=B_SPLINE_CURVE_WITH_KNOTS ( 'NONE', 3,
 ( #11098, #6645, #9432, #8511, #5715, #1771, #5658, #11284, #3677, #4740, #11340, #5531, #2688, #1029, #9306, #2759, #8330, #6461, #21, #7392, #7331, #4683, #2621, #10413, #6523, #1956, #2883, #9488, #1832, #4618, #3798, #8396, #6398, #10169, #7448, #5595, #12022, #9371 ),
 .UNSPECIFIED., .F., .F.,
 ( 4, 2, 2, 2, 2, 2, 2, 2, 2, 2, 2, 2, 2, 2, 2, 2, 2, 2, 4 ),
 ( 0.01596000347429163760, 0.01693787742768196672, 0.01791575138107229584, 0.01840468835776752285, 0.01889362533446274986, 0.01987149928785320388, 0.02084937324124365790, 0.02182724719463410845, 0.02280512114802456247, 0.02378299510141501649, 0.02476086905480547051, 0.02573874300819592453, 0.02671661696158637855, 0.02720555393828160556, 0.02769449091497682910, 0.02867236486836731088, 0.02965023882175778919, 0.03062811277514827096, 0.03160598672853875274 ),
 .UNSPECIFIED. ) ;
#11781=LINE ( 'NONE', #10900, #3174 ) ;
#11792=DIRECTION ( 'NONE',  ( -8.163404592832030268E-17, 1.000000000000000000, -0.000000000000000000 ) ) ;
#11795=AXIS2_PLACEMENT_3D ( 'NONE', #6210, #774, #642 ) ;
#11797=CARTESIAN_POINT ( 'NONE',  ( -22.49999999999997868, 24.00000000000001421, -126.4213562373092685 ) ) ;
#11800=ORIENTED_EDGE ( 'NONE', *, *, #2610, .F. ) ;
#11801=CARTESIAN_POINT ( 'NONE',  ( -925.0000000000000000, 101.9999999999999858, -124.6807709998038405 ) ) ;
#11803=EDGE_CURVE ( 'NONE', #7797, #11532, #8408, .T. ) ;
#11804=DIRECTION ( 'NONE',  ( -8.163404592832030268E-17, 1.000000000000000000, -0.000000000000000000 ) ) ;
#11806=DIRECTION ( 'NONE',  ( -0.000000000000000000, -0.000000000000000000, -1.000000000000000000 ) ) ;
#11811=CARTESIAN_POINT ( 'NONE',  ( -382.5120035867337265, 68.79460237993339433, -139.7124243609125642 ) ) ;
#11815=CARTESIAN_POINT ( 'NONE',  ( -371.4259950879257985, 104.0958151038622646, -140.9456086550797238 ) ) ;
#11817=CARTESIAN_POINT ( 'NONE',  ( -373.6571679095217746, 67.00567956805471681, -111.2964104634416174 ) ) ;
#11831=CARTESIAN_POINT ( 'NONE',  ( -270.0000000000000000, 139.9999999999999716, -126.4213562373076059 ) ) ;
#11834=ORIENTED_EDGE ( 'NONE', *, *, #11843, .T. ) ;
#11835=ADVANCED_FACE ( 'NONE', ( #297, #4082, #232, #8831, #5052, #4142, #4018, #7973, #3256, #2281, #7097 ), #5986, .F. ) ;
#11843=EDGE_CURVE ( 'NONE', #3288, #3585, #483, .T. ) ;
#11850=DIRECTION ( 'NONE',  ( -1.000000000000000000, 0.000000000000000000, 0.000000000000000000 ) ) ;
#11853=DIRECTION ( 'NONE',  ( 3.061276722312011504E-17, -1.000000000000000000, 0.000000000000000000 ) ) ;
#11855=CARTESIAN_POINT ( 'NONE',  ( -825.1278902672576123, 83.51360356663558093, -104.7380248171173918 ) ) ;
#11856=CARTESIAN_POINT ( 'NONE',  ( -379.1756773959688189, 62.02252057344967540, -123.5830889625225240 ) ) ;
#11858=CARTESIAN_POINT ( 'NONE',  ( -379.7921418149325063, 63.07164944986214294, -118.2218589047913611 ) ) ;
#11859=DIRECTION ( 'NONE',  ( 3.061276722312011504E-17, -1.000000000000000000, 0.000000000000000000 ) ) ;
#11861=CARTESIAN_POINT ( 'NONE',  ( -372.5553489903112450, 63.65594039108665925, -103.2085620308231313 ) ) ;
#11866=CARTESIAN_POINT ( 'NONE',  ( -372.5444667781683847, 101.5648799869878616, -129.1176400678176890 ) ) ;
#11869=FACE_OUTER_BOUND ( 'NONE', #10103, .T. ) ;
#11871=AXIS2_PLACEMENT_3D ( 'NONE', #9821, #9940, #10750 ) ;
#11875=ORIENTED_EDGE ( 'NONE', *, *, #9166, .T. ) ;
#11876=ORIENTED_EDGE ( 'NONE', *, *, #7214, .F. ) ;
#11878=AXIS2_PLACEMENT_3D ( 'NONE', #9646, #5689, #1128 ) ;
#11884=CARTESIAN_POINT ( 'NONE',  ( -379.2287960991276350, 101.8908318547082956, -122.2816696692770790 ) ) ;
#11900=ORIENTED_EDGE ( 'NONE', *, *, #3742, .T. ) ;
#11903=LINE ( 'NONE', #8403, #6681 ) ;
#11908=EDGE_LOOP ( 'NONE', ( #7574, #9297 ) ) ;
#11909=CARTESIAN_POINT ( 'NONE',  ( -828.7881391348988700, 78.01879388416006122, -144.2812265043193349 ) ) ;
#11920=DIRECTION ( 'NONE',  ( -8.163404592832030268E-17, 1.000000000000000000, -0.000000000000000000 ) ) ;
#11922=AXIS2_PLACEMENT_3D ( 'NONE', #8846, #8790, #4154 ) ;
#11927=CARTESIAN_POINT ( 'NONE',  ( -202.4999999999999716, 24.00000000000000711, -126.4213562373080180 ) ) ;
#11930=VECTOR ( 'NONE', #996, 1000.000000000000000 ) ;
#11938=EDGE_LOOP ( 'NONE', ( #2856, #379, #2220, #9803, #1318, #9897 ) ) ;
#11941=VECTOR ( 'NONE', #10283, 1000.000000000000000 ) ;
#11945=CARTESIAN_POINT ( 'NONE',  ( -372.4795512858445932, 62.20687173184607843, -127.6666720957034613 ) ) ;
#11957=AXIS2_PLACEMENT_3D ( 'NONE', #9048, #10904, #7955 ) ;
#11961=CARTESIAN_POINT ( 'NONE',  ( -142.5000000000000000, 152.0000000000000000, -126.4213562373084301 ) ) ;
#11969=EDGE_CURVE ( 'NONE', #7745, #11140, #8209, .T. ) ;
#11974=CARTESIAN_POINT ( 'NONE',  ( -821.5848584200502955, 74.20299736547755742, -143.0985335409774564 ) ) ;
#11975=ORIENTED_EDGE ( 'NONE', *, *, #12081, .F. ) ;
#11976=CARTESIAN_POINT ( 'NONE',  ( -370.3216402360161510, 56.83652478535064034, -116.0642080048412765 ) ) ;
#11984=CARTESIAN_POINT ( 'NONE',  ( -371.5518914047726753, 60.29737756751269728, -107.7881083410018590 ) ) ;
#11987=ORIENTED_EDGE ( 'NONE', *, *, #2285, .F. ) ;
#11993=CARTESIAN_POINT ( 'NONE',  ( -372.7918232332913817, 100.6587063813212524, -131.9323245634151647 ) ) ;
#11999=DIRECTION ( 'NONE',  ( -8.163404592832030268E-17, 1.000000000000000000, -0.000000000000000000 ) ) ;
#12006=ORIENTED_EDGE ( 'NONE', *, *, #8338, .F. ) ;
#12007=CARTESIAN_POINT ( 'NONE',  ( -379.3954710152061693, 62.38904131120219176, -128.6202947307455986 ) ) ;
#12018=CYLINDRICAL_SURFACE ( 'NONE', #7250, 7.500000000000007105 ) ;
#12021=ORIENTED_EDGE ( 'NONE', *, *, #2374, .F. ) ;
#12022=CARTESIAN_POINT ( 'NONE',  ( -818.8285638327207607, 79.00056486031988356, -144.4573442453747703 ) ) ;
#12034=CARTESIAN_POINT ( 'NONE',  ( -827.8143761345638723, 75.63828352384244624, -105.7174308425203861 ) ) ;
#12039=EDGE_CURVE ( 'NONE', #5834, #2997, #9112, .T. ) ;
#12055=CARTESIAN_POINT ( 'NONE',  ( -370.2276204871495224, 107.4109403250190553, -132.4627799267513240 ) ) ;
#12064=CARTESIAN_POINT ( 'NONE',  ( -381.3712298478259299, 97.88558035699080051, -136.8492573808261170 ) ) ;
#12071=VECTOR ( 'NONE', #5591, 1000.000000000000000 ) ;
#12077=CARTESIAN_POINT ( 'NONE',  ( -381.7589254172675055, 66.96601053460138075, -137.8868535322980904 ) ) ;
#12081=EDGE_CURVE ( 'NONE', #4125, #233, #9187, .T. ) ;
#12088=CARTESIAN_POINT ( 'NONE',  ( -150.0000000000000000, 152.0000000000000000, -126.4213562373084301 ) ) ;
#12090=AXIS2_PLACEMENT_3D ( 'NONE', #12088, #4420, #9174 ) ;
#12092=ORIENTED_EDGE ( 'NONE', *, *, #11550, .F. ) ;
#12095=DIRECTION ( 'NONE',  ( 0.000000000000000000, 1.000000000000000000, -0.000000000000000000 ) ) ;
#12100=CARTESIAN_POINT ( 'NONE',  ( -97.49999999999998579, -9.213203435596451385, -126.4213562373088564 ) ) ;
#12103=CARTESIAN_POINT ( 'NONE',  ( -819.8422515189663500, 75.63891865958716210, -105.7172146583290981 ) ) ;
#12106=ORIENTED_EDGE ( 'NONE', *, *, #2029, .T. ) ;
#12110=VERTEX_POINT ( 'NONE', #1834 ) ;
#12115=DIRECTION ( 'NONE',  ( -1.000000000000000000, 0.000000000000000000, 0.000000000000000000 ) ) ;
#12118=EDGE_CURVE ( 'NONE', #1615, #8369, #2806, .T. ) ;
#12133=CARTESIAN_POINT ( 'NONE',  ( -384.1738508217867434, 89.73612439111585104, -143.1700354454309547 ) ) ;
#12134=VERTEX_POINT ( 'NONE', #7803 ) ;
#12136=ORIENTED_EDGE ( 'NONE', *, *, #10312, .F. ) ;
#12140=EDGE_CURVE ( 'NONE', #7569, #8281, #9656, .T. ) ;
#12142=AXIS2_PLACEMENT_3D ( 'NONE', #5966, #10603, #1275 ) ;
#12144=ORIENTED_EDGE ( 'NONE', *, *, #10971, .T. ) ;
#12145=CARTESIAN_POINT ( 'NONE',  ( -373.2887456909239745, 65.34136874336766709, -135.8269615355799260 ) ) ;
#12148=DIRECTION ( 'NONE',  ( -1.000000000000000000, 0.000000000000000000, 0.000000000000000000 ) ) ;
#12150=AXIS2_PLACEMENT_3D ( 'NONE', #590, #6976, #10746 ) ;
#12168=DIRECTION ( 'NONE',  ( 0.000000000000000000, 1.000000000000000000, -0.000000000000000000 ) ) ;
#12171=CARTESIAN_POINT ( 'NONE',  ( -819.3334343865096798, 76.46102376401661616, -105.4605772031390813 ) ) ;
#12176=CARTESIAN_POINT ( 'NONE',  ( -373.4567406865983799, 67.35621697460008761, -149.6081567629417464 ) ) ;
#12177=CARTESIAN_POINT ( 'NONE',  ( -373.6140596466332227, 97.17021033344401815, -111.5627346061585570 ) ) ;
#12181=CIRCLE ( 'NONE', #7634, 69.99999999999998579 ) ;
#12196=ORIENTED_EDGE ( 'NONE', *, *, #3649, .F. ) ;
#12198=CIRCLE ( 'NONE', #6854, 7.500000000000007105 ) ;
#12199=ORIENTED_EDGE ( 'NONE', *, *, #120, .F. ) ;
#12203=CARTESIAN_POINT ( 'NONE',  ( -372.6621819111771288, 64.05756744580553175, -146.5841632647092183 ) ) ;
#12206=FACE_OUTER_BOUND ( 'NONE', #4349, .T. ) ;
#12210=CARTESIAN_POINT ( 'NONE',  ( -375.0000000000000000, 81.99999999999995737, -159.6807709998038547 ) ) ;
#12222=ADVANCED_FACE ( 'NONE', ( #3452 ), #1489, .F. ) ;
#12229=ADVANCED_FACE ( 'NONE', ( #5363 ), #4947, .F. ) ;
#12231=CARTESIAN_POINT ( 'NONE',  ( -828.5728621739501705, 77.06309091183271676, -105.2972035265138544 ) ) ;
#12234=CARTESIAN_POINT ( 'NONE',  ( -381.2061940965588747, 98.23031827135795879, -112.9896125472073010 ) ) ;
ENDSEC;
END-ISO-10303-21;
